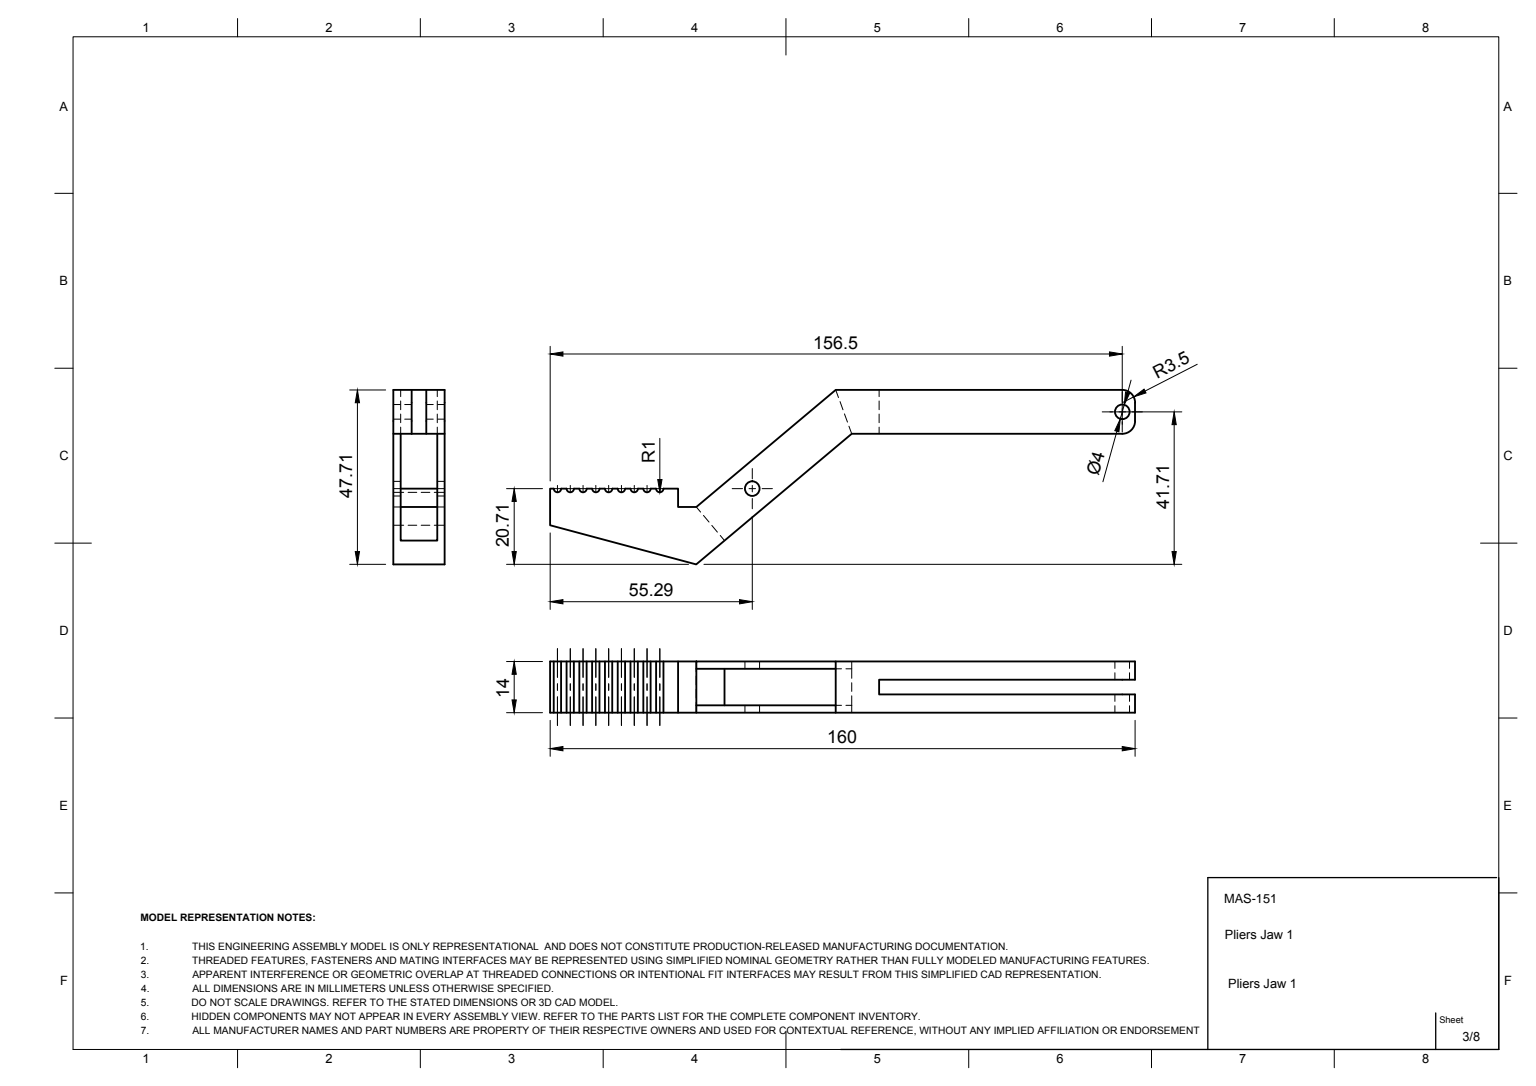
ISO-10303-21;
HEADER;
/* Generated by software containing ST-Developer
 * from STEP Tools, Inc. (www.steptools.com) 
 */

FILE_DESCRIPTION(
/* description */ ('STEP AP214'),
/* implementation_level */ '2;1');

FILE_NAME(
/* name */ 'Pliers Jaw 1.step',
/* time_stamp */ '2026-11-04T19:14:12-08:00',
/* author */ (''),
/* organization */ (''),
/* preprocessor_version */ 'ST-DEVELOPER v20.2',
/* originating_system */ 'Autodesk Translation Framework v15.17.0.0',
/* authorisation */ '');

FILE_SCHEMA (('AUTOMOTIVE_DESIGN { 1 0 10303 214 3 1 1 }'));
ENDSEC;

DATA;
#10=MECHANICAL_DESIGN_GEOMETRIC_PRESENTATION_REPRESENTATION('',(#99),#5990);
#85=SHAPE_REPRESENTATION_RELATIONSHIP('SRR','None',#6021,#92);
#92=ADVANCED_BREP_SHAPE_REPRESENTATION('',(#106),#5983);
#99=STYLED_ITEM('',(#6065),#106);
#106=MANIFOLD_SOLID_BREP('Body1',#3269);
#113=FACE_BOUND('',#427,.T.);
#114=FACE_BOUND('',#428,.T.);
#115=FACE_BOUND('',#430,.T.);
#116=FACE_BOUND('',#431,.T.);
#117=FACE_BOUND('',#463,.T.);
#118=FACE_BOUND('',#465,.T.);
#119=FACE_BOUND('',#467,.T.);
#120=FACE_BOUND('',#469,.T.);
#137=PLANE('',#3368);
#138=PLANE('',#3369);
#139=PLANE('',#3370);
#140=PLANE('',#3382);
#141=PLANE('',#3394);
#142=PLANE('',#3395);
#143=PLANE('',#3396);
#144=PLANE('',#3397);
#145=PLANE('',#3398);
#146=PLANE('',#3399);
#147=PLANE('',#3400);
#148=PLANE('',#3401);
#149=PLANE('',#3402);
#150=PLANE('',#3403);
#151=PLANE('',#3404);
#152=PLANE('',#3405);
#153=PLANE('',#3406);
#154=PLANE('',#3407);
#155=PLANE('',#3408);
#156=PLANE('',#3409);
#157=PLANE('',#3410);
#158=PLANE('',#3411);
#159=PLANE('',#3412);
#160=PLANE('',#3422);
#161=PLANE('',#3423);
#162=PLANE('',#3424);
#163=PLANE('',#3425);
#164=PLANE('',#3426);
#165=PLANE('',#3429);
#166=PLANE('',#3432);
#242=FACE_OUTER_BOUND('',#420,.T.);
#243=FACE_OUTER_BOUND('',#421,.T.);
#244=FACE_OUTER_BOUND('',#422,.T.);
#245=FACE_OUTER_BOUND('',#423,.T.);
#246=FACE_OUTER_BOUND('',#424,.T.);
#247=FACE_OUTER_BOUND('',#425,.T.);
#248=FACE_OUTER_BOUND('',#426,.T.);
#249=FACE_OUTER_BOUND('',#429,.T.);
#250=FACE_OUTER_BOUND('',#432,.T.);
#251=FACE_OUTER_BOUND('',#433,.T.);
#252=FACE_OUTER_BOUND('',#434,.T.);
#253=FACE_OUTER_BOUND('',#435,.T.);
#254=FACE_OUTER_BOUND('',#436,.T.);
#255=FACE_OUTER_BOUND('',#437,.T.);
#256=FACE_OUTER_BOUND('',#438,.T.);
#257=FACE_OUTER_BOUND('',#439,.T.);
#258=FACE_OUTER_BOUND('',#440,.T.);
#259=FACE_OUTER_BOUND('',#441,.T.);
#260=FACE_OUTER_BOUND('',#442,.T.);
#261=FACE_OUTER_BOUND('',#443,.T.);
#262=FACE_OUTER_BOUND('',#444,.T.);
#263=FACE_OUTER_BOUND('',#445,.T.);
#264=FACE_OUTER_BOUND('',#446,.T.);
#265=FACE_OUTER_BOUND('',#447,.T.);
#266=FACE_OUTER_BOUND('',#448,.T.);
#267=FACE_OUTER_BOUND('',#449,.T.);
#268=FACE_OUTER_BOUND('',#450,.T.);
#269=FACE_OUTER_BOUND('',#451,.T.);
#270=FACE_OUTER_BOUND('',#452,.T.);
#271=FACE_OUTER_BOUND('',#453,.T.);
#272=FACE_OUTER_BOUND('',#454,.T.);
#273=FACE_OUTER_BOUND('',#455,.T.);
#274=FACE_OUTER_BOUND('',#456,.T.);
#275=FACE_OUTER_BOUND('',#457,.T.);
#276=FACE_OUTER_BOUND('',#458,.T.);
#277=FACE_OUTER_BOUND('',#459,.T.);
#278=FACE_OUTER_BOUND('',#460,.T.);
#279=FACE_OUTER_BOUND('',#461,.T.);
#280=FACE_OUTER_BOUND('',#462,.T.);
#281=FACE_OUTER_BOUND('',#464,.T.);
#282=FACE_OUTER_BOUND('',#466,.T.);
#283=FACE_OUTER_BOUND('',#468,.T.);
#284=FACE_OUTER_BOUND('',#470,.T.);
#285=FACE_OUTER_BOUND('',#471,.T.);
#286=FACE_OUTER_BOUND('',#472,.T.);
#287=FACE_OUTER_BOUND('',#473,.T.);
#288=FACE_OUTER_BOUND('',#474,.T.);
#420=EDGE_LOOP('',(#2110,#2111,#2112,#2113));
#421=EDGE_LOOP('',(#2114,#2115,#2116,#2117));
#422=EDGE_LOOP('',(#2118,#2119,#2120,#2121));
#423=EDGE_LOOP('',(#2122,#2123,#2124,#2125));
#424=EDGE_LOOP('',(#2126,#2127,#2128,#2129));
#425=EDGE_LOOP('',(#2130,#2131,#2132,#2133));
#426=EDGE_LOOP('',(#2134,#2135,#2136,#2137,#2138,#2139,#2140,#2141,#2142,
#2143,#2144,#2145,#2146,#2147,#2148,#2149,#2150,#2151,#2152,#2153,#2154,
#2155,#2156,#2157,#2158,#2159,#2160,#2161,#2162,#2163));
#427=EDGE_LOOP('',(#2164));
#428=EDGE_LOOP('',(#2165));
#429=EDGE_LOOP('',(#2166,#2167,#2168,#2169,#2170,#2171,#2172,#2173,#2174,
#2175,#2176,#2177,#2178,#2179,#2180,#2181,#2182,#2183,#2184,#2185,#2186,
#2187,#2188,#2189,#2190,#2191,#2192,#2193,#2194,#2195));
#430=EDGE_LOOP('',(#2196));
#431=EDGE_LOOP('',(#2197));
#432=EDGE_LOOP('',(#2198,#2199,#2200,#2201));
#433=EDGE_LOOP('',(#2202,#2203,#2204,#2205));
#434=EDGE_LOOP('',(#2206,#2207,#2208,#2209));
#435=EDGE_LOOP('',(#2210,#2211,#2212,#2213));
#436=EDGE_LOOP('',(#2214,#2215,#2216,#2217));
#437=EDGE_LOOP('',(#2218,#2219,#2220,#2221));
#438=EDGE_LOOP('',(#2222,#2223,#2224,#2225));
#439=EDGE_LOOP('',(#2226,#2227,#2228,#2229));
#440=EDGE_LOOP('',(#2230,#2231,#2232,#2233));
#441=EDGE_LOOP('',(#2234,#2235,#2236,#2237,#2238,#2239));
#442=EDGE_LOOP('',(#2240,#2241,#2242,#2243));
#443=EDGE_LOOP('',(#2244,#2245,#2246,#2247));
#444=EDGE_LOOP('',(#2248,#2249,#2250,#2251));
#445=EDGE_LOOP('',(#2252,#2253,#2254,#2255,#2256,#2257,#2258,#2259));
#446=EDGE_LOOP('',(#2260,#2261,#2262,#2263,#2264,#2265,#2266,#2267,#2268,
#2269));
#447=EDGE_LOOP('',(#2270,#2271,#2272,#2273));
#448=EDGE_LOOP('',(#2274,#2275,#2276,#2277,#2278,#2279,#2280,#2281,#2282,
#2283));
#449=EDGE_LOOP('',(#2284,#2285,#2286,#2287));
#450=EDGE_LOOP('',(#2288,#2289,#2290,#2291));
#451=EDGE_LOOP('',(#2292,#2293,#2294,#2295));
#452=EDGE_LOOP('',(#2296,#2297,#2298,#2299));
#453=EDGE_LOOP('',(#2300,#2301,#2302,#2303));
#454=EDGE_LOOP('',(#2304,#2305,#2306,#2307));
#455=EDGE_LOOP('',(#2308,#2309,#2310,#2311));
#456=EDGE_LOOP('',(#2312,#2313,#2314,#2315));
#457=EDGE_LOOP('',(#2316,#2317,#2318,#2319));
#458=EDGE_LOOP('',(#2320,#2321,#2322,#2323));
#459=EDGE_LOOP('',(#2324,#2325,#2326,#2327));
#460=EDGE_LOOP('',(#2328,#2329,#2330,#2331));
#461=EDGE_LOOP('',(#2332,#2333,#2334,#2335));
#462=EDGE_LOOP('',(#2336,#2337,#2338,#2339));
#463=EDGE_LOOP('',(#2340));
#464=EDGE_LOOP('',(#2341,#2342,#2343,#2344));
#465=EDGE_LOOP('',(#2345));
#466=EDGE_LOOP('',(#2346,#2347,#2348,#2349,#2350,#2351));
#467=EDGE_LOOP('',(#2352));
#468=EDGE_LOOP('',(#2353,#2354,#2355,#2356,#2357,#2358));
#469=EDGE_LOOP('',(#2359));
#470=EDGE_LOOP('',(#2360,#2361,#2362,#2363));
#471=EDGE_LOOP('',(#2364,#2365,#2366,#2367));
#472=EDGE_LOOP('',(#2368,#2369,#2370,#2371));
#473=EDGE_LOOP('',(#2372,#2373,#2374,#2375));
#474=EDGE_LOOP('',(#2376,#2377,#2378,#2379));
#622=LINE('',#4656,#925);
#623=LINE('',#4662,#926);
#624=LINE('',#4668,#927);
#625=LINE('',#4674,#928);
#626=LINE('',#4679,#929);
#627=LINE('',#4681,#930);
#628=LINE('',#4683,#931);
#629=LINE('',#4684,#932);
#630=LINE('',#4688,#933);
#631=LINE('',#4690,#934);
#632=LINE('',#4692,#935);
#633=LINE('',#4693,#936);
#634=LINE('',#4697,#937);
#635=LINE('',#4701,#938);
#636=LINE('',#4703,#939);
#637=LINE('',#4705,#940);
#638=LINE('',#4707,#941);
#639=LINE('',#4709,#942);
#640=LINE('',#4713,#943);
#641=LINE('',#4717,#944);
#642=LINE('',#4721,#945);
#643=LINE('',#4725,#946);
#644=LINE('',#4729,#947);
#645=LINE('',#4733,#948);
#646=LINE('',#4737,#949);
#647=LINE('',#4741,#950);
#648=LINE('',#4745,#951);
#649=LINE('',#4747,#952);
#650=LINE('',#4749,#953);
#651=LINE('',#4751,#954);
#652=LINE('',#4753,#955);
#653=LINE('',#4757,#956);
#654=LINE('',#4762,#957);
#655=LINE('',#4764,#958);
#656=LINE('',#4766,#959);
#657=LINE('',#4768,#960);
#658=LINE('',#4770,#961);
#659=LINE('',#4774,#962);
#660=LINE('',#4778,#963);
#661=LINE('',#4782,#964);
#662=LINE('',#4786,#965);
#663=LINE('',#4790,#966);
#664=LINE('',#4794,#967);
#665=LINE('',#4798,#968);
#666=LINE('',#4802,#969);
#667=LINE('',#4806,#970);
#668=LINE('',#4808,#971);
#669=LINE('',#4809,#972);
#670=LINE('',#4811,#973);
#671=LINE('',#4812,#974);
#672=LINE('',#4814,#975);
#673=LINE('',#4815,#976);
#674=LINE('',#4817,#977);
#675=LINE('',#4818,#978);
#676=LINE('',#4820,#979);
#677=LINE('',#4821,#980);
#678=LINE('',#4823,#981);
#679=LINE('',#4824,#982);
#680=LINE('',#4826,#983);
#681=LINE('',#4827,#984);
#682=LINE('',#4829,#985);
#683=LINE('',#4830,#986);
#684=LINE('',#4832,#987);
#685=LINE('',#4833,#988);
#686=LINE('',#4835,#989);
#687=LINE('',#4836,#990);
#688=LINE('',#4838,#991);
#689=LINE('',#4840,#992);
#690=LINE('',#4841,#993);
#691=LINE('',#4844,#994);
#692=LINE('',#4845,#995);
#693=LINE('',#4847,#996);
#694=LINE('',#4848,#997);
#695=LINE('',#4850,#998);
#696=LINE('',#4854,#999);
#697=LINE('',#4856,#1000);
#698=LINE('',#4857,#1001);
#699=LINE('',#4859,#1002);
#700=LINE('',#4860,#1003);
#701=LINE('',#4864,#1004);
#702=LINE('',#4865,#1005);
#703=LINE('',#4866,#1006);
#704=LINE('',#4868,#1007);
#705=LINE('',#4870,#1008);
#706=LINE('',#4871,#1009);
#707=LINE('',#4875,#1010);
#708=LINE('',#4876,#1011);
#709=LINE('',#4877,#1012);
#710=LINE('',#4880,#1013);
#711=LINE('',#4882,#1014);
#712=LINE('',#4884,#1015);
#713=LINE('',#4886,#1016);
#714=LINE('',#4887,#1017);
#715=LINE('',#4888,#1018);
#716=LINE('',#4891,#1019);
#717=LINE('',#4902,#1020);
#718=LINE('',#4903,#1021);
#719=LINE('',#4905,#1022);
#720=LINE('',#4906,#1023);
#721=LINE('',#4912,#1024);
#722=LINE('',#4915,#1025);
#925=VECTOR('',#3693,2.);
#926=VECTOR('',#3700,2.);
#927=VECTOR('',#3707,2.);
#928=VECTOR('',#3714,2.);
#929=VECTOR('',#3719,1000.);
#930=VECTOR('',#3720,1000.);
#931=VECTOR('',#3721,1000.);
#932=VECTOR('',#3722,1000.);
#933=VECTOR('',#3725,1000.);
#934=VECTOR('',#3726,1000.);
#935=VECTOR('',#3727,1000.);
#936=VECTOR('',#3728,1000.);
#937=VECTOR('',#3731,1000.);
#938=VECTOR('',#3734,1000.);
#939=VECTOR('',#3735,1000.);
#940=VECTOR('',#3736,1000.);
#941=VECTOR('',#3737,1000.);
#942=VECTOR('',#3738,1000.);
#943=VECTOR('',#3741,1000.);
#944=VECTOR('',#3744,1000.);
#945=VECTOR('',#3747,1000.);
#946=VECTOR('',#3750,1000.);
#947=VECTOR('',#3753,1000.);
#948=VECTOR('',#3756,1000.);
#949=VECTOR('',#3759,1000.);
#950=VECTOR('',#3762,1000.);
#951=VECTOR('',#3765,1000.);
#952=VECTOR('',#3766,1000.);
#953=VECTOR('',#3767,1000.);
#954=VECTOR('',#3768,1000.);
#955=VECTOR('',#3769,1000.);
#956=VECTOR('',#3774,1000.);
#957=VECTOR('',#3779,1000.);
#958=VECTOR('',#3780,1000.);
#959=VECTOR('',#3781,1000.);
#960=VECTOR('',#3782,1000.);
#961=VECTOR('',#3783,1000.);
#962=VECTOR('',#3786,1000.);
#963=VECTOR('',#3789,1000.);
#964=VECTOR('',#3792,1000.);
#965=VECTOR('',#3795,1000.);
#966=VECTOR('',#3798,1000.);
#967=VECTOR('',#3801,1000.);
#968=VECTOR('',#3804,1000.);
#969=VECTOR('',#3807,1000.);
#970=VECTOR('',#3810,1000.);
#971=VECTOR('',#3811,1000.);
#972=VECTOR('',#3812,1000.);
#973=VECTOR('',#3815,1000.);
#974=VECTOR('',#3816,1000.);
#975=VECTOR('',#3819,1000.);
#976=VECTOR('',#3820,1000.);
#977=VECTOR('',#3823,1000.);
#978=VECTOR('',#3824,1000.);
#979=VECTOR('',#3827,1000.);
#980=VECTOR('',#3828,1000.);
#981=VECTOR('',#3831,1000.);
#982=VECTOR('',#3832,1000.);
#983=VECTOR('',#3835,1000.);
#984=VECTOR('',#3836,1000.);
#985=VECTOR('',#3839,1000.);
#986=VECTOR('',#3840,1000.);
#987=VECTOR('',#3843,1000.);
#988=VECTOR('',#3844,1000.);
#989=VECTOR('',#3847,1000.);
#990=VECTOR('',#3848,1000.);
#991=VECTOR('',#3851,1000.);
#992=VECTOR('',#3852,1000.);
#993=VECTOR('',#3853,1000.);
#994=VECTOR('',#3856,1000.);
#995=VECTOR('',#3857,1000.);
#996=VECTOR('',#3860,1000.);
#997=VECTOR('',#3861,1000.);
#998=VECTOR('',#3864,1000.);
#999=VECTOR('',#3867,1000.);
#1000=VECTOR('',#3868,1000.);
#1001=VECTOR('',#3869,1000.);
#1002=VECTOR('',#3870,1000.);
#1003=VECTOR('',#3871,1000.);
#1004=VECTOR('',#3874,1000.);
#1005=VECTOR('',#3875,1000.);
#1006=VECTOR('',#3876,1000.);
#1007=VECTOR('',#3877,1000.);
#1008=VECTOR('',#3878,1000.);
#1009=VECTOR('',#3879,1000.);
#1010=VECTOR('',#3882,1000.);
#1011=VECTOR('',#3883,1000.);
#1012=VECTOR('',#3884,1000.);
#1013=VECTOR('',#3887,1000.);
#1014=VECTOR('',#3888,1000.);
#1015=VECTOR('',#3889,1000.);
#1016=VECTOR('',#3890,1000.);
#1017=VECTOR('',#3891,1000.);
#1018=VECTOR('',#3892,1000.);
#1019=VECTOR('',#3897,1000.);
#1020=VECTOR('',#3918,1000.);
#1021=VECTOR('',#3919,1000.);
#1022=VECTOR('',#3922,1000.);
#1023=VECTOR('',#3923,1000.);
#1024=VECTOR('',#3934,1000.);
#1025=VECTOR('',#3939,1000.);
#1228=CIRCLE('',#3357,2.);
#1229=CIRCLE('',#3358,2.);
#1230=CIRCLE('',#3360,2.);
#1231=CIRCLE('',#3361,2.);
#1232=CIRCLE('',#3363,2.);
#1233=CIRCLE('',#3364,2.);
#1234=CIRCLE('',#3366,2.);
#1235=CIRCLE('',#3367,2.);
#1236=CIRCLE('',#3371,3.5);
#1237=CIRCLE('',#3372,1.);
#1238=CIRCLE('',#3373,1.);
#1239=CIRCLE('',#3374,1.);
#1240=CIRCLE('',#3375,1.);
#1241=CIRCLE('',#3376,1.);
#1242=CIRCLE('',#3377,1.);
#1243=CIRCLE('',#3378,1.);
#1244=CIRCLE('',#3379,1.);
#1245=CIRCLE('',#3380,1.);
#1246=CIRCLE('',#3381,3.5);
#1247=CIRCLE('',#3383,3.5);
#1248=CIRCLE('',#3384,3.5);
#1249=CIRCLE('',#3385,1.);
#1250=CIRCLE('',#3386,1.);
#1251=CIRCLE('',#3387,1.);
#1252=CIRCLE('',#3388,1.);
#1253=CIRCLE('',#3389,1.);
#1254=CIRCLE('',#3390,1.);
#1255=CIRCLE('',#3391,1.);
#1256=CIRCLE('',#3392,1.);
#1257=CIRCLE('',#3393,1.);
#1258=CIRCLE('',#3427,3.5);
#1259=CIRCLE('',#3428,3.5);
#1260=CIRCLE('',#3430,3.5);
#1261=CIRCLE('',#3431,3.5);
#1356=VERTEX_POINT('',#4653);
#1357=VERTEX_POINT('',#4655);
#1358=VERTEX_POINT('',#4659);
#1359=VERTEX_POINT('',#4661);
#1360=VERTEX_POINT('',#4665);
#1361=VERTEX_POINT('',#4667);
#1362=VERTEX_POINT('',#4671);
#1363=VERTEX_POINT('',#4673);
#1364=VERTEX_POINT('',#4677);
#1365=VERTEX_POINT('',#4678);
#1366=VERTEX_POINT('',#4680);
#1367=VERTEX_POINT('',#4682);
#1368=VERTEX_POINT('',#4686);
#1369=VERTEX_POINT('',#4687);
#1370=VERTEX_POINT('',#4689);
#1371=VERTEX_POINT('',#4691);
#1372=VERTEX_POINT('',#4695);
#1373=VERTEX_POINT('',#4696);
#1374=VERTEX_POINT('',#4698);
#1375=VERTEX_POINT('',#4700);
#1376=VERTEX_POINT('',#4702);
#1377=VERTEX_POINT('',#4704);
#1378=VERTEX_POINT('',#4706);
#1379=VERTEX_POINT('',#4708);
#1380=VERTEX_POINT('',#4710);
#1381=VERTEX_POINT('',#4712);
#1382=VERTEX_POINT('',#4714);
#1383=VERTEX_POINT('',#4716);
#1384=VERTEX_POINT('',#4718);
#1385=VERTEX_POINT('',#4720);
#1386=VERTEX_POINT('',#4722);
#1387=VERTEX_POINT('',#4724);
#1388=VERTEX_POINT('',#4726);
#1389=VERTEX_POINT('',#4728);
#1390=VERTEX_POINT('',#4730);
#1391=VERTEX_POINT('',#4732);
#1392=VERTEX_POINT('',#4734);
#1393=VERTEX_POINT('',#4736);
#1394=VERTEX_POINT('',#4738);
#1395=VERTEX_POINT('',#4740);
#1396=VERTEX_POINT('',#4742);
#1397=VERTEX_POINT('',#4744);
#1398=VERTEX_POINT('',#4746);
#1399=VERTEX_POINT('',#4748);
#1400=VERTEX_POINT('',#4750);
#1401=VERTEX_POINT('',#4752);
#1402=VERTEX_POINT('',#4756);
#1403=VERTEX_POINT('',#4759);
#1404=VERTEX_POINT('',#4761);
#1405=VERTEX_POINT('',#4763);
#1406=VERTEX_POINT('',#4765);
#1407=VERTEX_POINT('',#4767);
#1408=VERTEX_POINT('',#4769);
#1409=VERTEX_POINT('',#4771);
#1410=VERTEX_POINT('',#4773);
#1411=VERTEX_POINT('',#4775);
#1412=VERTEX_POINT('',#4777);
#1413=VERTEX_POINT('',#4779);
#1414=VERTEX_POINT('',#4781);
#1415=VERTEX_POINT('',#4783);
#1416=VERTEX_POINT('',#4785);
#1417=VERTEX_POINT('',#4787);
#1418=VERTEX_POINT('',#4789);
#1419=VERTEX_POINT('',#4791);
#1420=VERTEX_POINT('',#4793);
#1421=VERTEX_POINT('',#4795);
#1422=VERTEX_POINT('',#4797);
#1423=VERTEX_POINT('',#4799);
#1424=VERTEX_POINT('',#4801);
#1425=VERTEX_POINT('',#4803);
#1426=VERTEX_POINT('',#4805);
#1427=VERTEX_POINT('',#4807);
#1428=VERTEX_POINT('',#4839);
#1429=VERTEX_POINT('',#4843);
#1430=VERTEX_POINT('',#4852);
#1431=VERTEX_POINT('',#4853);
#1432=VERTEX_POINT('',#4855);
#1433=VERTEX_POINT('',#4858);
#1434=VERTEX_POINT('',#4862);
#1435=VERTEX_POINT('',#4863);
#1436=VERTEX_POINT('',#4867);
#1437=VERTEX_POINT('',#4869);
#1438=VERTEX_POINT('',#4873);
#1439=VERTEX_POINT('',#4874);
#1440=VERTEX_POINT('',#4879);
#1441=VERTEX_POINT('',#4881);
#1442=VERTEX_POINT('',#4883);
#1443=VERTEX_POINT('',#4885);
#1651=EDGE_CURVE('',#1356,#1356,#1228,.T.);
#1652=EDGE_CURVE('',#1356,#1357,#622,.T.);
#1653=EDGE_CURVE('',#1357,#1357,#1229,.T.);
#1654=EDGE_CURVE('',#1358,#1358,#1230,.T.);
#1655=EDGE_CURVE('',#1358,#1359,#623,.T.);
#1656=EDGE_CURVE('',#1359,#1359,#1231,.T.);
#1657=EDGE_CURVE('',#1360,#1360,#1232,.T.);
#1658=EDGE_CURVE('',#1360,#1361,#624,.T.);
#1659=EDGE_CURVE('',#1361,#1361,#1233,.T.);
#1660=EDGE_CURVE('',#1362,#1362,#1234,.T.);
#1661=EDGE_CURVE('',#1362,#1363,#625,.T.);
#1662=EDGE_CURVE('',#1363,#1363,#1235,.T.);
#1663=EDGE_CURVE('',#1364,#1365,#626,.T.);
#1664=EDGE_CURVE('',#1365,#1366,#627,.T.);
#1665=EDGE_CURVE('',#1366,#1367,#628,.T.);
#1666=EDGE_CURVE('',#1367,#1364,#629,.T.);
#1667=EDGE_CURVE('',#1368,#1369,#630,.T.);
#1668=EDGE_CURVE('',#1368,#1370,#631,.T.);
#1669=EDGE_CURVE('',#1370,#1371,#632,.T.);
#1670=EDGE_CURVE('',#1369,#1371,#633,.T.);
#1671=EDGE_CURVE('',#1372,#1373,#634,.T.);
#1672=EDGE_CURVE('',#1373,#1374,#1236,.T.);
#1673=EDGE_CURVE('',#1374,#1375,#635,.T.);
#1674=EDGE_CURVE('',#1375,#1376,#636,.T.);
#1675=EDGE_CURVE('',#1376,#1377,#637,.T.);
#1676=EDGE_CURVE('',#1377,#1378,#638,.T.);
#1677=EDGE_CURVE('',#1378,#1379,#639,.T.);
#1678=EDGE_CURVE('',#1380,#1379,#1237,.T.);
#1679=EDGE_CURVE('',#1380,#1381,#640,.T.);
#1680=EDGE_CURVE('',#1382,#1381,#1238,.T.);
#1681=EDGE_CURVE('',#1382,#1383,#641,.T.);
#1682=EDGE_CURVE('',#1384,#1383,#1239,.T.);
#1683=EDGE_CURVE('',#1384,#1385,#642,.T.);
#1684=EDGE_CURVE('',#1386,#1385,#1240,.T.);
#1685=EDGE_CURVE('',#1386,#1387,#643,.T.);
#1686=EDGE_CURVE('',#1388,#1387,#1241,.T.);
#1687=EDGE_CURVE('',#1388,#1389,#644,.T.);
#1688=EDGE_CURVE('',#1390,#1389,#1242,.T.);
#1689=EDGE_CURVE('',#1390,#1391,#645,.T.);
#1690=EDGE_CURVE('',#1392,#1391,#1243,.T.);
#1691=EDGE_CURVE('',#1392,#1393,#646,.T.);
#1692=EDGE_CURVE('',#1394,#1393,#1244,.T.);
#1693=EDGE_CURVE('',#1394,#1395,#647,.T.);
#1694=EDGE_CURVE('',#1396,#1395,#1245,.T.);
#1695=EDGE_CURVE('',#1396,#1397,#648,.T.);
#1696=EDGE_CURVE('',#1397,#1398,#649,.T.);
#1697=EDGE_CURVE('',#1398,#1399,#650,.T.);
#1698=EDGE_CURVE('',#1399,#1400,#651,.T.);
#1699=EDGE_CURVE('',#1400,#1401,#652,.T.);
#1700=EDGE_CURVE('',#1401,#1372,#1246,.T.);
#1701=EDGE_CURVE('',#1402,#1370,#653,.T.);
#1702=EDGE_CURVE('',#1402,#1365,#1247,.T.);
#1703=EDGE_CURVE('',#1364,#1403,#1248,.T.);
#1704=EDGE_CURVE('',#1404,#1403,#654,.T.);
#1705=EDGE_CURVE('',#1405,#1404,#655,.T.);
#1706=EDGE_CURVE('',#1406,#1405,#656,.T.);
#1707=EDGE_CURVE('',#1407,#1406,#657,.T.);
#1708=EDGE_CURVE('',#1408,#1407,#658,.T.);
#1709=EDGE_CURVE('',#1408,#1409,#1249,.T.);
#1710=EDGE_CURVE('',#1410,#1409,#659,.T.);
#1711=EDGE_CURVE('',#1410,#1411,#1250,.T.);
#1712=EDGE_CURVE('',#1412,#1411,#660,.T.);
#1713=EDGE_CURVE('',#1412,#1413,#1251,.T.);
#1714=EDGE_CURVE('',#1414,#1413,#661,.T.);
#1715=EDGE_CURVE('',#1414,#1415,#1252,.T.);
#1716=EDGE_CURVE('',#1416,#1415,#662,.T.);
#1717=EDGE_CURVE('',#1416,#1417,#1253,.T.);
#1718=EDGE_CURVE('',#1418,#1417,#663,.T.);
#1719=EDGE_CURVE('',#1418,#1419,#1254,.T.);
#1720=EDGE_CURVE('',#1420,#1419,#664,.T.);
#1721=EDGE_CURVE('',#1420,#1421,#1255,.T.);
#1722=EDGE_CURVE('',#1422,#1421,#665,.T.);
#1723=EDGE_CURVE('',#1422,#1423,#1256,.T.);
#1724=EDGE_CURVE('',#1424,#1423,#666,.T.);
#1725=EDGE_CURVE('',#1424,#1425,#1257,.T.);
#1726=EDGE_CURVE('',#1426,#1425,#667,.T.);
#1727=EDGE_CURVE('',#1427,#1426,#668,.T.);
#1728=EDGE_CURVE('',#1371,#1427,#669,.T.);
#1729=EDGE_CURVE('',#1411,#1393,#670,.T.);
#1730=EDGE_CURVE('',#1392,#1412,#671,.T.);
#1731=EDGE_CURVE('',#1413,#1391,#672,.T.);
#1732=EDGE_CURVE('',#1390,#1414,#673,.T.);
#1733=EDGE_CURVE('',#1415,#1389,#674,.T.);
#1734=EDGE_CURVE('',#1388,#1416,#675,.T.);
#1735=EDGE_CURVE('',#1417,#1387,#676,.T.);
#1736=EDGE_CURVE('',#1386,#1418,#677,.T.);
#1737=EDGE_CURVE('',#1419,#1385,#678,.T.);
#1738=EDGE_CURVE('',#1384,#1420,#679,.T.);
#1739=EDGE_CURVE('',#1421,#1383,#680,.T.);
#1740=EDGE_CURVE('',#1382,#1422,#681,.T.);
#1741=EDGE_CURVE('',#1423,#1381,#682,.T.);
#1742=EDGE_CURVE('',#1380,#1424,#683,.T.);
#1743=EDGE_CURVE('',#1425,#1379,#684,.T.);
#1744=EDGE_CURVE('',#1378,#1426,#685,.T.);
#1745=EDGE_CURVE('',#1394,#1410,#686,.T.);
#1746=EDGE_CURVE('',#1409,#1395,#687,.T.);
#1747=EDGE_CURVE('',#1377,#1427,#688,.T.);
#1748=EDGE_CURVE('',#1376,#1428,#689,.T.);
#1749=EDGE_CURVE('',#1369,#1428,#690,.T.);
#1750=EDGE_CURVE('',#1375,#1429,#691,.T.);
#1751=EDGE_CURVE('',#1429,#1428,#692,.T.);
#1752=EDGE_CURVE('',#1398,#1406,#693,.T.);
#1753=EDGE_CURVE('',#1397,#1407,#694,.T.);
#1754=EDGE_CURVE('',#1399,#1405,#695,.T.);
#1755=EDGE_CURVE('',#1430,#1431,#696,.T.);
#1756=EDGE_CURVE('',#1431,#1432,#697,.T.);
#1757=EDGE_CURVE('',#1400,#1432,#698,.T.);
#1758=EDGE_CURVE('',#1433,#1404,#699,.T.);
#1759=EDGE_CURVE('',#1430,#1433,#700,.T.);
#1760=EDGE_CURVE('',#1434,#1435,#701,.T.);
#1761=EDGE_CURVE('',#1435,#1401,#702,.T.);
#1762=EDGE_CURVE('',#1433,#1432,#703,.T.);
#1763=EDGE_CURVE('',#1403,#1436,#704,.T.);
#1764=EDGE_CURVE('',#1437,#1436,#705,.T.);
#1765=EDGE_CURVE('',#1434,#1437,#706,.T.);
#1766=EDGE_CURVE('',#1438,#1439,#707,.T.);
#1767=EDGE_CURVE('',#1438,#1373,#708,.T.);
#1768=EDGE_CURVE('',#1372,#1439,#709,.T.);
#1769=EDGE_CURVE('',#1374,#1440,#710,.T.);
#1770=EDGE_CURVE('',#1440,#1441,#711,.T.);
#1771=EDGE_CURVE('',#1442,#1441,#712,.T.);
#1772=EDGE_CURVE('',#1443,#1442,#713,.T.);
#1773=EDGE_CURVE('',#1443,#1402,#714,.T.);
#1774=EDGE_CURVE('',#1368,#1429,#715,.T.);
#1775=EDGE_CURVE('',#1396,#1408,#716,.T.);
#1776=EDGE_CURVE('',#1432,#1429,#717,.T.);
#1777=EDGE_CURVE('',#1433,#1368,#718,.T.);
#1778=EDGE_CURVE('',#1428,#1431,#719,.T.);
#1779=EDGE_CURVE('',#1369,#1430,#720,.T.);
#1780=EDGE_CURVE('',#1440,#1438,#1258,.T.);
#1781=EDGE_CURVE('',#1439,#1435,#1259,.T.);
#1782=EDGE_CURVE('',#1441,#1434,#721,.T.);
#1783=EDGE_CURVE('',#1366,#1443,#1260,.T.);
#1784=EDGE_CURVE('',#1442,#1437,#722,.T.);
#1785=EDGE_CURVE('',#1436,#1367,#1261,.T.);
#2110=ORIENTED_EDGE('',*,*,#1651,.F.);
#2111=ORIENTED_EDGE('',*,*,#1652,.T.);
#2112=ORIENTED_EDGE('',*,*,#1653,.F.);
#2113=ORIENTED_EDGE('',*,*,#1652,.F.);
#2114=ORIENTED_EDGE('',*,*,#1654,.T.);
#2115=ORIENTED_EDGE('',*,*,#1655,.T.);
#2116=ORIENTED_EDGE('',*,*,#1656,.T.);
#2117=ORIENTED_EDGE('',*,*,#1655,.F.);
#2118=ORIENTED_EDGE('',*,*,#1657,.F.);
#2119=ORIENTED_EDGE('',*,*,#1658,.T.);
#2120=ORIENTED_EDGE('',*,*,#1659,.T.);
#2121=ORIENTED_EDGE('',*,*,#1658,.F.);
#2122=ORIENTED_EDGE('',*,*,#1660,.F.);
#2123=ORIENTED_EDGE('',*,*,#1661,.T.);
#2124=ORIENTED_EDGE('',*,*,#1662,.T.);
#2125=ORIENTED_EDGE('',*,*,#1661,.F.);
#2126=ORIENTED_EDGE('',*,*,#1663,.T.);
#2127=ORIENTED_EDGE('',*,*,#1664,.T.);
#2128=ORIENTED_EDGE('',*,*,#1665,.T.);
#2129=ORIENTED_EDGE('',*,*,#1666,.T.);
#2130=ORIENTED_EDGE('',*,*,#1667,.F.);
#2131=ORIENTED_EDGE('',*,*,#1668,.T.);
#2132=ORIENTED_EDGE('',*,*,#1669,.T.);
#2133=ORIENTED_EDGE('',*,*,#1670,.F.);
#2134=ORIENTED_EDGE('',*,*,#1671,.T.);
#2135=ORIENTED_EDGE('',*,*,#1672,.T.);
#2136=ORIENTED_EDGE('',*,*,#1673,.T.);
#2137=ORIENTED_EDGE('',*,*,#1674,.T.);
#2138=ORIENTED_EDGE('',*,*,#1675,.T.);
#2139=ORIENTED_EDGE('',*,*,#1676,.T.);
#2140=ORIENTED_EDGE('',*,*,#1677,.T.);
#2141=ORIENTED_EDGE('',*,*,#1678,.F.);
#2142=ORIENTED_EDGE('',*,*,#1679,.T.);
#2143=ORIENTED_EDGE('',*,*,#1680,.F.);
#2144=ORIENTED_EDGE('',*,*,#1681,.T.);
#2145=ORIENTED_EDGE('',*,*,#1682,.F.);
#2146=ORIENTED_EDGE('',*,*,#1683,.T.);
#2147=ORIENTED_EDGE('',*,*,#1684,.F.);
#2148=ORIENTED_EDGE('',*,*,#1685,.T.);
#2149=ORIENTED_EDGE('',*,*,#1686,.F.);
#2150=ORIENTED_EDGE('',*,*,#1687,.T.);
#2151=ORIENTED_EDGE('',*,*,#1688,.F.);
#2152=ORIENTED_EDGE('',*,*,#1689,.T.);
#2153=ORIENTED_EDGE('',*,*,#1690,.F.);
#2154=ORIENTED_EDGE('',*,*,#1691,.T.);
#2155=ORIENTED_EDGE('',*,*,#1692,.F.);
#2156=ORIENTED_EDGE('',*,*,#1693,.T.);
#2157=ORIENTED_EDGE('',*,*,#1694,.F.);
#2158=ORIENTED_EDGE('',*,*,#1695,.T.);
#2159=ORIENTED_EDGE('',*,*,#1696,.T.);
#2160=ORIENTED_EDGE('',*,*,#1697,.T.);
#2161=ORIENTED_EDGE('',*,*,#1698,.T.);
#2162=ORIENTED_EDGE('',*,*,#1699,.T.);
#2163=ORIENTED_EDGE('',*,*,#1700,.T.);
#2164=ORIENTED_EDGE('',*,*,#1651,.T.);
#2165=ORIENTED_EDGE('',*,*,#1662,.F.);
#2166=ORIENTED_EDGE('',*,*,#1701,.F.);
#2167=ORIENTED_EDGE('',*,*,#1702,.T.);
#2168=ORIENTED_EDGE('',*,*,#1663,.F.);
#2169=ORIENTED_EDGE('',*,*,#1703,.T.);
#2170=ORIENTED_EDGE('',*,*,#1704,.F.);
#2171=ORIENTED_EDGE('',*,*,#1705,.F.);
#2172=ORIENTED_EDGE('',*,*,#1706,.F.);
#2173=ORIENTED_EDGE('',*,*,#1707,.F.);
#2174=ORIENTED_EDGE('',*,*,#1708,.F.);
#2175=ORIENTED_EDGE('',*,*,#1709,.T.);
#2176=ORIENTED_EDGE('',*,*,#1710,.F.);
#2177=ORIENTED_EDGE('',*,*,#1711,.T.);
#2178=ORIENTED_EDGE('',*,*,#1712,.F.);
#2179=ORIENTED_EDGE('',*,*,#1713,.T.);
#2180=ORIENTED_EDGE('',*,*,#1714,.F.);
#2181=ORIENTED_EDGE('',*,*,#1715,.T.);
#2182=ORIENTED_EDGE('',*,*,#1716,.F.);
#2183=ORIENTED_EDGE('',*,*,#1717,.T.);
#2184=ORIENTED_EDGE('',*,*,#1718,.F.);
#2185=ORIENTED_EDGE('',*,*,#1719,.T.);
#2186=ORIENTED_EDGE('',*,*,#1720,.F.);
#2187=ORIENTED_EDGE('',*,*,#1721,.T.);
#2188=ORIENTED_EDGE('',*,*,#1722,.F.);
#2189=ORIENTED_EDGE('',*,*,#1723,.T.);
#2190=ORIENTED_EDGE('',*,*,#1724,.F.);
#2191=ORIENTED_EDGE('',*,*,#1725,.T.);
#2192=ORIENTED_EDGE('',*,*,#1726,.F.);
#2193=ORIENTED_EDGE('',*,*,#1727,.F.);
#2194=ORIENTED_EDGE('',*,*,#1728,.F.);
#2195=ORIENTED_EDGE('',*,*,#1669,.F.);
#2196=ORIENTED_EDGE('',*,*,#1656,.F.);
#2197=ORIENTED_EDGE('',*,*,#1657,.T.);
#2198=ORIENTED_EDGE('',*,*,#1712,.T.);
#2199=ORIENTED_EDGE('',*,*,#1729,.T.);
#2200=ORIENTED_EDGE('',*,*,#1691,.F.);
#2201=ORIENTED_EDGE('',*,*,#1730,.T.);
#2202=ORIENTED_EDGE('',*,*,#1714,.T.);
#2203=ORIENTED_EDGE('',*,*,#1731,.T.);
#2204=ORIENTED_EDGE('',*,*,#1689,.F.);
#2205=ORIENTED_EDGE('',*,*,#1732,.T.);
#2206=ORIENTED_EDGE('',*,*,#1716,.T.);
#2207=ORIENTED_EDGE('',*,*,#1733,.T.);
#2208=ORIENTED_EDGE('',*,*,#1687,.F.);
#2209=ORIENTED_EDGE('',*,*,#1734,.T.);
#2210=ORIENTED_EDGE('',*,*,#1718,.T.);
#2211=ORIENTED_EDGE('',*,*,#1735,.T.);
#2212=ORIENTED_EDGE('',*,*,#1685,.F.);
#2213=ORIENTED_EDGE('',*,*,#1736,.T.);
#2214=ORIENTED_EDGE('',*,*,#1720,.T.);
#2215=ORIENTED_EDGE('',*,*,#1737,.T.);
#2216=ORIENTED_EDGE('',*,*,#1683,.F.);
#2217=ORIENTED_EDGE('',*,*,#1738,.T.);
#2218=ORIENTED_EDGE('',*,*,#1722,.T.);
#2219=ORIENTED_EDGE('',*,*,#1739,.T.);
#2220=ORIENTED_EDGE('',*,*,#1681,.F.);
#2221=ORIENTED_EDGE('',*,*,#1740,.T.);
#2222=ORIENTED_EDGE('',*,*,#1724,.T.);
#2223=ORIENTED_EDGE('',*,*,#1741,.T.);
#2224=ORIENTED_EDGE('',*,*,#1679,.F.);
#2225=ORIENTED_EDGE('',*,*,#1742,.T.);
#2226=ORIENTED_EDGE('',*,*,#1726,.T.);
#2227=ORIENTED_EDGE('',*,*,#1743,.T.);
#2228=ORIENTED_EDGE('',*,*,#1677,.F.);
#2229=ORIENTED_EDGE('',*,*,#1744,.T.);
#2230=ORIENTED_EDGE('',*,*,#1693,.F.);
#2231=ORIENTED_EDGE('',*,*,#1745,.T.);
#2232=ORIENTED_EDGE('',*,*,#1710,.T.);
#2233=ORIENTED_EDGE('',*,*,#1746,.T.);
#2234=ORIENTED_EDGE('',*,*,#1747,.F.);
#2235=ORIENTED_EDGE('',*,*,#1675,.F.);
#2236=ORIENTED_EDGE('',*,*,#1748,.T.);
#2237=ORIENTED_EDGE('',*,*,#1749,.F.);
#2238=ORIENTED_EDGE('',*,*,#1670,.T.);
#2239=ORIENTED_EDGE('',*,*,#1728,.T.);
#2240=ORIENTED_EDGE('',*,*,#1750,.T.);
#2241=ORIENTED_EDGE('',*,*,#1751,.T.);
#2242=ORIENTED_EDGE('',*,*,#1748,.F.);
#2243=ORIENTED_EDGE('',*,*,#1674,.F.);
#2244=ORIENTED_EDGE('',*,*,#1707,.T.);
#2245=ORIENTED_EDGE('',*,*,#1752,.F.);
#2246=ORIENTED_EDGE('',*,*,#1696,.F.);
#2247=ORIENTED_EDGE('',*,*,#1753,.T.);
#2248=ORIENTED_EDGE('',*,*,#1706,.T.);
#2249=ORIENTED_EDGE('',*,*,#1754,.F.);
#2250=ORIENTED_EDGE('',*,*,#1697,.F.);
#2251=ORIENTED_EDGE('',*,*,#1752,.T.);
#2252=ORIENTED_EDGE('',*,*,#1755,.T.);
#2253=ORIENTED_EDGE('',*,*,#1756,.T.);
#2254=ORIENTED_EDGE('',*,*,#1757,.F.);
#2255=ORIENTED_EDGE('',*,*,#1698,.F.);
#2256=ORIENTED_EDGE('',*,*,#1754,.T.);
#2257=ORIENTED_EDGE('',*,*,#1705,.T.);
#2258=ORIENTED_EDGE('',*,*,#1758,.F.);
#2259=ORIENTED_EDGE('',*,*,#1759,.F.);
#2260=ORIENTED_EDGE('',*,*,#1760,.T.);
#2261=ORIENTED_EDGE('',*,*,#1761,.T.);
#2262=ORIENTED_EDGE('',*,*,#1699,.F.);
#2263=ORIENTED_EDGE('',*,*,#1757,.T.);
#2264=ORIENTED_EDGE('',*,*,#1762,.F.);
#2265=ORIENTED_EDGE('',*,*,#1758,.T.);
#2266=ORIENTED_EDGE('',*,*,#1704,.T.);
#2267=ORIENTED_EDGE('',*,*,#1763,.T.);
#2268=ORIENTED_EDGE('',*,*,#1764,.F.);
#2269=ORIENTED_EDGE('',*,*,#1765,.F.);
#2270=ORIENTED_EDGE('',*,*,#1766,.F.);
#2271=ORIENTED_EDGE('',*,*,#1767,.T.);
#2272=ORIENTED_EDGE('',*,*,#1671,.F.);
#2273=ORIENTED_EDGE('',*,*,#1768,.T.);
#2274=ORIENTED_EDGE('',*,*,#1673,.F.);
#2275=ORIENTED_EDGE('',*,*,#1769,.T.);
#2276=ORIENTED_EDGE('',*,*,#1770,.T.);
#2277=ORIENTED_EDGE('',*,*,#1771,.F.);
#2278=ORIENTED_EDGE('',*,*,#1772,.F.);
#2279=ORIENTED_EDGE('',*,*,#1773,.T.);
#2280=ORIENTED_EDGE('',*,*,#1701,.T.);
#2281=ORIENTED_EDGE('',*,*,#1668,.F.);
#2282=ORIENTED_EDGE('',*,*,#1774,.T.);
#2283=ORIENTED_EDGE('',*,*,#1750,.F.);
#2284=ORIENTED_EDGE('',*,*,#1727,.T.);
#2285=ORIENTED_EDGE('',*,*,#1744,.F.);
#2286=ORIENTED_EDGE('',*,*,#1676,.F.);
#2287=ORIENTED_EDGE('',*,*,#1747,.T.);
#2288=ORIENTED_EDGE('',*,*,#1695,.F.);
#2289=ORIENTED_EDGE('',*,*,#1775,.T.);
#2290=ORIENTED_EDGE('',*,*,#1708,.T.);
#2291=ORIENTED_EDGE('',*,*,#1753,.F.);
#2292=ORIENTED_EDGE('',*,*,#1709,.F.);
#2293=ORIENTED_EDGE('',*,*,#1775,.F.);
#2294=ORIENTED_EDGE('',*,*,#1694,.T.);
#2295=ORIENTED_EDGE('',*,*,#1746,.F.);
#2296=ORIENTED_EDGE('',*,*,#1725,.F.);
#2297=ORIENTED_EDGE('',*,*,#1742,.F.);
#2298=ORIENTED_EDGE('',*,*,#1678,.T.);
#2299=ORIENTED_EDGE('',*,*,#1743,.F.);
#2300=ORIENTED_EDGE('',*,*,#1723,.F.);
#2301=ORIENTED_EDGE('',*,*,#1740,.F.);
#2302=ORIENTED_EDGE('',*,*,#1680,.T.);
#2303=ORIENTED_EDGE('',*,*,#1741,.F.);
#2304=ORIENTED_EDGE('',*,*,#1721,.F.);
#2305=ORIENTED_EDGE('',*,*,#1738,.F.);
#2306=ORIENTED_EDGE('',*,*,#1682,.T.);
#2307=ORIENTED_EDGE('',*,*,#1739,.F.);
#2308=ORIENTED_EDGE('',*,*,#1719,.F.);
#2309=ORIENTED_EDGE('',*,*,#1736,.F.);
#2310=ORIENTED_EDGE('',*,*,#1684,.T.);
#2311=ORIENTED_EDGE('',*,*,#1737,.F.);
#2312=ORIENTED_EDGE('',*,*,#1717,.F.);
#2313=ORIENTED_EDGE('',*,*,#1734,.F.);
#2314=ORIENTED_EDGE('',*,*,#1686,.T.);
#2315=ORIENTED_EDGE('',*,*,#1735,.F.);
#2316=ORIENTED_EDGE('',*,*,#1715,.F.);
#2317=ORIENTED_EDGE('',*,*,#1732,.F.);
#2318=ORIENTED_EDGE('',*,*,#1688,.T.);
#2319=ORIENTED_EDGE('',*,*,#1733,.F.);
#2320=ORIENTED_EDGE('',*,*,#1713,.F.);
#2321=ORIENTED_EDGE('',*,*,#1730,.F.);
#2322=ORIENTED_EDGE('',*,*,#1690,.T.);
#2323=ORIENTED_EDGE('',*,*,#1731,.F.);
#2324=ORIENTED_EDGE('',*,*,#1711,.F.);
#2325=ORIENTED_EDGE('',*,*,#1745,.F.);
#2326=ORIENTED_EDGE('',*,*,#1692,.T.);
#2327=ORIENTED_EDGE('',*,*,#1729,.F.);
#2328=ORIENTED_EDGE('',*,*,#1776,.T.);
#2329=ORIENTED_EDGE('',*,*,#1774,.F.);
#2330=ORIENTED_EDGE('',*,*,#1777,.F.);
#2331=ORIENTED_EDGE('',*,*,#1762,.T.);
#2332=ORIENTED_EDGE('',*,*,#1778,.T.);
#2333=ORIENTED_EDGE('',*,*,#1755,.F.);
#2334=ORIENTED_EDGE('',*,*,#1779,.F.);
#2335=ORIENTED_EDGE('',*,*,#1749,.T.);
#2336=ORIENTED_EDGE('',*,*,#1667,.T.);
#2337=ORIENTED_EDGE('',*,*,#1779,.T.);
#2338=ORIENTED_EDGE('',*,*,#1759,.T.);
#2339=ORIENTED_EDGE('',*,*,#1777,.T.);
#2340=ORIENTED_EDGE('',*,*,#1659,.F.);
#2341=ORIENTED_EDGE('',*,*,#1751,.F.);
#2342=ORIENTED_EDGE('',*,*,#1776,.F.);
#2343=ORIENTED_EDGE('',*,*,#1756,.F.);
#2344=ORIENTED_EDGE('',*,*,#1778,.F.);
#2345=ORIENTED_EDGE('',*,*,#1660,.T.);
#2346=ORIENTED_EDGE('',*,*,#1770,.F.);
#2347=ORIENTED_EDGE('',*,*,#1780,.T.);
#2348=ORIENTED_EDGE('',*,*,#1766,.T.);
#2349=ORIENTED_EDGE('',*,*,#1781,.T.);
#2350=ORIENTED_EDGE('',*,*,#1760,.F.);
#2351=ORIENTED_EDGE('',*,*,#1782,.F.);
#2352=ORIENTED_EDGE('',*,*,#1653,.T.);
#2353=ORIENTED_EDGE('',*,*,#1665,.F.);
#2354=ORIENTED_EDGE('',*,*,#1783,.T.);
#2355=ORIENTED_EDGE('',*,*,#1772,.T.);
#2356=ORIENTED_EDGE('',*,*,#1784,.T.);
#2357=ORIENTED_EDGE('',*,*,#1764,.T.);
#2358=ORIENTED_EDGE('',*,*,#1785,.T.);
#2359=ORIENTED_EDGE('',*,*,#1654,.F.);
#2360=ORIENTED_EDGE('',*,*,#1765,.T.);
#2361=ORIENTED_EDGE('',*,*,#1784,.F.);
#2362=ORIENTED_EDGE('',*,*,#1771,.T.);
#2363=ORIENTED_EDGE('',*,*,#1782,.T.);
#2364=ORIENTED_EDGE('',*,*,#1672,.F.);
#2365=ORIENTED_EDGE('',*,*,#1767,.F.);
#2366=ORIENTED_EDGE('',*,*,#1780,.F.);
#2367=ORIENTED_EDGE('',*,*,#1769,.F.);
#2368=ORIENTED_EDGE('',*,*,#1783,.F.);
#2369=ORIENTED_EDGE('',*,*,#1664,.F.);
#2370=ORIENTED_EDGE('',*,*,#1702,.F.);
#2371=ORIENTED_EDGE('',*,*,#1773,.F.);
#2372=ORIENTED_EDGE('',*,*,#1700,.F.);
#2373=ORIENTED_EDGE('',*,*,#1761,.F.);
#2374=ORIENTED_EDGE('',*,*,#1781,.F.);
#2375=ORIENTED_EDGE('',*,*,#1768,.F.);
#2376=ORIENTED_EDGE('',*,*,#1785,.F.);
#2377=ORIENTED_EDGE('',*,*,#1763,.F.);
#2378=ORIENTED_EDGE('',*,*,#1703,.F.);
#2379=ORIENTED_EDGE('',*,*,#1666,.F.);
#3028=CYLINDRICAL_SURFACE('',#3356,2.);
#3029=CYLINDRICAL_SURFACE('',#3359,2.);
#3030=CYLINDRICAL_SURFACE('',#3362,2.);
#3031=CYLINDRICAL_SURFACE('',#3365,2.);
#3032=CYLINDRICAL_SURFACE('',#3413,1.);
#3033=CYLINDRICAL_SURFACE('',#3414,1.);
#3034=CYLINDRICAL_SURFACE('',#3415,1.);
#3035=CYLINDRICAL_SURFACE('',#3416,1.);
#3036=CYLINDRICAL_SURFACE('',#3417,1.);
#3037=CYLINDRICAL_SURFACE('',#3418,1.);
#3038=CYLINDRICAL_SURFACE('',#3419,1.);
#3039=CYLINDRICAL_SURFACE('',#3420,1.);
#3040=CYLINDRICAL_SURFACE('',#3421,1.);
#3041=CYLINDRICAL_SURFACE('',#3433,3.5);
#3042=CYLINDRICAL_SURFACE('',#3434,3.5);
#3043=CYLINDRICAL_SURFACE('',#3435,3.5);
#3044=CYLINDRICAL_SURFACE('',#3436,3.5);
#3091=ADVANCED_FACE('',(#242),#3028,.F.);
#3092=ADVANCED_FACE('',(#243),#3029,.F.);
#3093=ADVANCED_FACE('',(#244),#3030,.F.);
#3094=ADVANCED_FACE('',(#245),#3031,.F.);
#3095=ADVANCED_FACE('',(#246),#137,.F.);
#3096=ADVANCED_FACE('',(#247),#138,.F.);
#3097=ADVANCED_FACE('',(#248,#113,#114),#139,.F.);
#3098=ADVANCED_FACE('',(#249,#115,#116),#140,.T.);
#3099=ADVANCED_FACE('',(#250),#141,.F.);
#3100=ADVANCED_FACE('',(#251),#142,.F.);
#3101=ADVANCED_FACE('',(#252),#143,.F.);
#3102=ADVANCED_FACE('',(#253),#144,.F.);
#3103=ADVANCED_FACE('',(#254),#145,.F.);
#3104=ADVANCED_FACE('',(#255),#146,.F.);
#3105=ADVANCED_FACE('',(#256),#147,.F.);
#3106=ADVANCED_FACE('',(#257),#148,.F.);
#3107=ADVANCED_FACE('',(#258),#149,.F.);
#3108=ADVANCED_FACE('',(#259),#150,.F.);
#3109=ADVANCED_FACE('',(#260),#151,.F.);
#3110=ADVANCED_FACE('',(#261),#152,.F.);
#3111=ADVANCED_FACE('',(#262),#153,.F.);
#3112=ADVANCED_FACE('',(#263),#154,.F.);
#3113=ADVANCED_FACE('',(#264),#155,.F.);
#3114=ADVANCED_FACE('',(#265),#156,.F.);
#3115=ADVANCED_FACE('',(#266),#157,.F.);
#3116=ADVANCED_FACE('',(#267),#158,.F.);
#3117=ADVANCED_FACE('',(#268),#159,.F.);
#3118=ADVANCED_FACE('',(#269),#3032,.F.);
#3119=ADVANCED_FACE('',(#270),#3033,.F.);
#3120=ADVANCED_FACE('',(#271),#3034,.F.);
#3121=ADVANCED_FACE('',(#272),#3035,.F.);
#3122=ADVANCED_FACE('',(#273),#3036,.F.);
#3123=ADVANCED_FACE('',(#274),#3037,.F.);
#3124=ADVANCED_FACE('',(#275),#3038,.F.);
#3125=ADVANCED_FACE('',(#276),#3039,.F.);
#3126=ADVANCED_FACE('',(#277),#3040,.F.);
#3127=ADVANCED_FACE('',(#278),#160,.F.);
#3128=ADVANCED_FACE('',(#279),#161,.F.);
#3129=ADVANCED_FACE('',(#280,#117),#162,.T.);
#3130=ADVANCED_FACE('',(#281,#118),#163,.F.);
#3131=ADVANCED_FACE('',(#282,#119),#164,.F.);
#3132=ADVANCED_FACE('',(#283,#120),#165,.T.);
#3133=ADVANCED_FACE('',(#284),#166,.T.);
#3134=ADVANCED_FACE('',(#285),#3041,.T.);
#3135=ADVANCED_FACE('',(#286),#3042,.T.);
#3136=ADVANCED_FACE('',(#287),#3043,.T.);
#3137=ADVANCED_FACE('',(#288),#3044,.T.);
#3269=CLOSED_SHELL('',(#3091,#3092,#3093,#3094,#3095,#3096,#3097,#3098,
#3099,#3100,#3101,#3102,#3103,#3104,#3105,#3106,#3107,#3108,#3109,#3110,
#3111,#3112,#3113,#3114,#3115,#3116,#3117,#3118,#3119,#3120,#3121,#3122,
#3123,#3124,#3125,#3126,#3127,#3128,#3129,#3130,#3131,#3132,#3133,#3134,
#3135,#3136,#3137));
#3355=AXIS2_PLACEMENT_3D('',#4651,#3687,#3688);
#3356=AXIS2_PLACEMENT_3D('',#4652,#3689,#3690);
#3357=AXIS2_PLACEMENT_3D('',#4654,#3691,#3692);
#3358=AXIS2_PLACEMENT_3D('',#4657,#3694,#3695);
#3359=AXIS2_PLACEMENT_3D('',#4658,#3696,#3697);
#3360=AXIS2_PLACEMENT_3D('',#4660,#3698,#3699);
#3361=AXIS2_PLACEMENT_3D('',#4663,#3701,#3702);
#3362=AXIS2_PLACEMENT_3D('',#4664,#3703,#3704);
#3363=AXIS2_PLACEMENT_3D('',#4666,#3705,#3706);
#3364=AXIS2_PLACEMENT_3D('',#4669,#3708,#3709);
#3365=AXIS2_PLACEMENT_3D('',#4670,#3710,#3711);
#3366=AXIS2_PLACEMENT_3D('',#4672,#3712,#3713);
#3367=AXIS2_PLACEMENT_3D('',#4675,#3715,#3716);
#3368=AXIS2_PLACEMENT_3D('',#4676,#3717,#3718);
#3369=AXIS2_PLACEMENT_3D('',#4685,#3723,#3724);
#3370=AXIS2_PLACEMENT_3D('',#4694,#3729,#3730);
#3371=AXIS2_PLACEMENT_3D('',#4699,#3732,#3733);
#3372=AXIS2_PLACEMENT_3D('',#4711,#3739,#3740);
#3373=AXIS2_PLACEMENT_3D('',#4715,#3742,#3743);
#3374=AXIS2_PLACEMENT_3D('',#4719,#3745,#3746);
#3375=AXIS2_PLACEMENT_3D('',#4723,#3748,#3749);
#3376=AXIS2_PLACEMENT_3D('',#4727,#3751,#3752);
#3377=AXIS2_PLACEMENT_3D('',#4731,#3754,#3755);
#3378=AXIS2_PLACEMENT_3D('',#4735,#3757,#3758);
#3379=AXIS2_PLACEMENT_3D('',#4739,#3760,#3761);
#3380=AXIS2_PLACEMENT_3D('',#4743,#3763,#3764);
#3381=AXIS2_PLACEMENT_3D('',#4754,#3770,#3771);
#3382=AXIS2_PLACEMENT_3D('',#4755,#3772,#3773);
#3383=AXIS2_PLACEMENT_3D('',#4758,#3775,#3776);
#3384=AXIS2_PLACEMENT_3D('',#4760,#3777,#3778);
#3385=AXIS2_PLACEMENT_3D('',#4772,#3784,#3785);
#3386=AXIS2_PLACEMENT_3D('',#4776,#3787,#3788);
#3387=AXIS2_PLACEMENT_3D('',#4780,#3790,#3791);
#3388=AXIS2_PLACEMENT_3D('',#4784,#3793,#3794);
#3389=AXIS2_PLACEMENT_3D('',#4788,#3796,#3797);
#3390=AXIS2_PLACEMENT_3D('',#4792,#3799,#3800);
#3391=AXIS2_PLACEMENT_3D('',#4796,#3802,#3803);
#3392=AXIS2_PLACEMENT_3D('',#4800,#3805,#3806);
#3393=AXIS2_PLACEMENT_3D('',#4804,#3808,#3809);
#3394=AXIS2_PLACEMENT_3D('',#4810,#3813,#3814);
#3395=AXIS2_PLACEMENT_3D('',#4813,#3817,#3818);
#3396=AXIS2_PLACEMENT_3D('',#4816,#3821,#3822);
#3397=AXIS2_PLACEMENT_3D('',#4819,#3825,#3826);
#3398=AXIS2_PLACEMENT_3D('',#4822,#3829,#3830);
#3399=AXIS2_PLACEMENT_3D('',#4825,#3833,#3834);
#3400=AXIS2_PLACEMENT_3D('',#4828,#3837,#3838);
#3401=AXIS2_PLACEMENT_3D('',#4831,#3841,#3842);
#3402=AXIS2_PLACEMENT_3D('',#4834,#3845,#3846);
#3403=AXIS2_PLACEMENT_3D('',#4837,#3849,#3850);
#3404=AXIS2_PLACEMENT_3D('',#4842,#3854,#3855);
#3405=AXIS2_PLACEMENT_3D('',#4846,#3858,#3859);
#3406=AXIS2_PLACEMENT_3D('',#4849,#3862,#3863);
#3407=AXIS2_PLACEMENT_3D('',#4851,#3865,#3866);
#3408=AXIS2_PLACEMENT_3D('',#4861,#3872,#3873);
#3409=AXIS2_PLACEMENT_3D('',#4872,#3880,#3881);
#3410=AXIS2_PLACEMENT_3D('',#4878,#3885,#3886);
#3411=AXIS2_PLACEMENT_3D('',#4889,#3893,#3894);
#3412=AXIS2_PLACEMENT_3D('',#4890,#3895,#3896);
#3413=AXIS2_PLACEMENT_3D('',#4892,#3898,#3899);
#3414=AXIS2_PLACEMENT_3D('',#4893,#3900,#3901);
#3415=AXIS2_PLACEMENT_3D('',#4894,#3902,#3903);
#3416=AXIS2_PLACEMENT_3D('',#4895,#3904,#3905);
#3417=AXIS2_PLACEMENT_3D('',#4896,#3906,#3907);
#3418=AXIS2_PLACEMENT_3D('',#4897,#3908,#3909);
#3419=AXIS2_PLACEMENT_3D('',#4898,#3910,#3911);
#3420=AXIS2_PLACEMENT_3D('',#4899,#3912,#3913);
#3421=AXIS2_PLACEMENT_3D('',#4900,#3914,#3915);
#3422=AXIS2_PLACEMENT_3D('',#4901,#3916,#3917);
#3423=AXIS2_PLACEMENT_3D('',#4904,#3920,#3921);
#3424=AXIS2_PLACEMENT_3D('',#4907,#3924,#3925);
#3425=AXIS2_PLACEMENT_3D('',#4908,#3926,#3927);
#3426=AXIS2_PLACEMENT_3D('',#4909,#3928,#3929);
#3427=AXIS2_PLACEMENT_3D('',#4910,#3930,#3931);
#3428=AXIS2_PLACEMENT_3D('',#4911,#3932,#3933);
#3429=AXIS2_PLACEMENT_3D('',#4913,#3935,#3936);
#3430=AXIS2_PLACEMENT_3D('',#4914,#3937,#3938);
#3431=AXIS2_PLACEMENT_3D('',#4916,#3940,#3941);
#3432=AXIS2_PLACEMENT_3D('',#4917,#3942,#3943);
#3433=AXIS2_PLACEMENT_3D('',#4918,#3944,#3945);
#3434=AXIS2_PLACEMENT_3D('',#4919,#3946,#3947);
#3435=AXIS2_PLACEMENT_3D('',#4920,#3948,#3949);
#3436=AXIS2_PLACEMENT_3D('',#4921,#3950,#3951);
#3687=DIRECTION('axis',(0.,0.,1.));
#3688=DIRECTION('refdir',(1.,0.,0.));
#3689=DIRECTION('center_axis',(0.,0.,-1.));
#3690=DIRECTION('ref_axis',(-1.,0.,0.));
#3691=DIRECTION('center_axis',(0.,0.,-1.));
#3692=DIRECTION('ref_axis',(-1.,0.,0.));
#3693=DIRECTION('',(0.,0.,-1.));
#3694=DIRECTION('center_axis',(5.55111512312578E-17,2.47817639425258E-17,
1.));
#3695=DIRECTION('ref_axis',(1.,-1.37566424599088E-33,-5.55111512312578E-17));
#3696=DIRECTION('center_axis',(0.,0.,-1.));
#3697=DIRECTION('ref_axis',(-1.,0.,0.));
#3698=DIRECTION('center_axis',(5.55111512312578E-17,2.47817639425258E-17,
1.));
#3699=DIRECTION('ref_axis',(1.,-1.37566424599088E-33,-5.55111512312578E-17));
#3700=DIRECTION('',(0.,0.,-1.));
#3701=DIRECTION('center_axis',(0.,0.,-1.));
#3702=DIRECTION('ref_axis',(-1.,0.,0.));
#3703=DIRECTION('center_axis',(0.,0.,1.));
#3704=DIRECTION('ref_axis',(1.,0.,0.));
#3705=DIRECTION('center_axis',(0.,0.,1.));
#3706=DIRECTION('ref_axis',(1.,0.,0.));
#3707=DIRECTION('',(0.,0.,1.));
#3708=DIRECTION('center_axis',(0.,0.,1.));
#3709=DIRECTION('ref_axis',(1.,0.,0.));
#3710=DIRECTION('center_axis',(0.,0.,1.));
#3711=DIRECTION('ref_axis',(1.,0.,0.));
#3712=DIRECTION('center_axis',(0.,0.,1.));
#3713=DIRECTION('ref_axis',(1.,0.,0.));
#3714=DIRECTION('',(0.,0.,1.));
#3715=DIRECTION('center_axis',(0.,0.,1.));
#3716=DIRECTION('ref_axis',(1.,0.,0.));
#3717=DIRECTION('center_axis',(0.,1.,0.));
#3718=DIRECTION('ref_axis',(0.,0.,1.));
#3719=DIRECTION('',(1.,0.,0.));
#3720=DIRECTION('',(0.,0.,1.));
#3721=DIRECTION('',(-1.,1.79745021839835E-17,5.55111512312578E-17));
#3722=DIRECTION('',(0.,0.,-1.));
#3723=DIRECTION('center_axis',(-0.766044443118972,-0.642787609686546,0.));
#3724=DIRECTION('ref_axis',(0.642787609686546,-0.766044443118972,0.));
#3725=DIRECTION('',(-0.642787609686546,0.766044443118972,0.));
#3726=DIRECTION('',(0.,0.,-1.));
#3727=DIRECTION('',(-0.642787609686546,0.766044443118972,0.));
#3728=DIRECTION('',(0.,0.,-1.));
#3729=DIRECTION('center_axis',(0.,0.,-1.));
#3730=DIRECTION('ref_axis',(-1.,0.,0.));
#3731=DIRECTION('',(1.,0.,0.));
#3732=DIRECTION('center_axis',(0.,0.,1.));
#3733=DIRECTION('ref_axis',(-1.,0.,0.));
#3734=DIRECTION('',(-8.47613560090905E-17,1.,0.));
#3735=DIRECTION('',(-0.642787609686546,0.766044443118972,0.));
#3736=DIRECTION('',(0.,1.,0.));
#3737=DIRECTION('',(1.,0.,0.));
#3738=DIRECTION('',(-1.23908819712629E-16,1.,0.));
#3739=DIRECTION('center_axis',(0.,0.,1.));
#3740=DIRECTION('ref_axis',(1.,0.,0.));
#3741=DIRECTION('',(-1.23908819712629E-16,1.,0.));
#3742=DIRECTION('center_axis',(0.,0.,1.));
#3743=DIRECTION('ref_axis',(1.,0.,0.));
#3744=DIRECTION('',(-1.23908819712629E-16,1.,0.));
#3745=DIRECTION('center_axis',(0.,0.,1.));
#3746=DIRECTION('ref_axis',(1.,0.,0.));
#3747=DIRECTION('',(-1.23908819712629E-16,1.,0.));
#3748=DIRECTION('center_axis',(0.,0.,1.));
#3749=DIRECTION('ref_axis',(1.,0.,0.));
#3750=DIRECTION('',(-1.23908819712629E-16,1.,0.));
#3751=DIRECTION('center_axis',(0.,0.,1.));
#3752=DIRECTION('ref_axis',(1.,0.,0.));
#3753=DIRECTION('',(-1.23908819712629E-16,1.,0.));
#3754=DIRECTION('center_axis',(0.,0.,1.));
#3755=DIRECTION('ref_axis',(1.,0.,0.));
#3756=DIRECTION('',(-1.23908819712629E-16,1.,0.));
#3757=DIRECTION('center_axis',(0.,0.,1.));
#3758=DIRECTION('ref_axis',(1.,0.,0.));
#3759=DIRECTION('',(-1.23908819712629E-16,1.,0.));
#3760=DIRECTION('center_axis',(0.,0.,1.));
#3761=DIRECTION('ref_axis',(1.,0.,0.));
#3762=DIRECTION('',(-1.23908819712629E-16,1.,0.));
#3763=DIRECTION('center_axis',(0.,0.,1.));
#3764=DIRECTION('ref_axis',(1.,0.,0.));
#3765=DIRECTION('',(-1.23908819712629E-16,1.,0.));
#3766=DIRECTION('',(-1.,0.,0.));
#3767=DIRECTION('',(-0.258819045102514,-0.96592582628907,0.));
#3768=DIRECTION('',(0.642787609686546,-0.766044443118972,0.));
#3769=DIRECTION('',(-4.47692281884469E-17,-1.,0.));
#3770=DIRECTION('center_axis',(0.,0.,1.));
#3771=DIRECTION('ref_axis',(-1.,0.,0.));
#3772=DIRECTION('center_axis',(0.,0.,-1.));
#3773=DIRECTION('ref_axis',(-1.,0.,0.));
#3774=DIRECTION('',(-8.47613560090905E-17,1.,0.));
#3775=DIRECTION('center_axis',(0.,0.,-1.));
#3776=DIRECTION('ref_axis',(-1.,0.,0.));
#3777=DIRECTION('center_axis',(0.,0.,-1.));
#3778=DIRECTION('ref_axis',(-1.,0.,0.));
#3779=DIRECTION('',(-4.47692281884469E-17,-1.,0.));
#3780=DIRECTION('',(0.642787609686546,-0.766044443118972,0.));
#3781=DIRECTION('',(-0.258819045102514,-0.96592582628907,0.));
#3782=DIRECTION('',(-1.,0.,0.));
#3783=DIRECTION('',(-1.23908819712629E-16,1.,0.));
#3784=DIRECTION('center_axis',(0.,0.,1.));
#3785=DIRECTION('ref_axis',(1.,0.,0.));
#3786=DIRECTION('',(-1.23908819712629E-16,1.,0.));
#3787=DIRECTION('center_axis',(0.,0.,1.));
#3788=DIRECTION('ref_axis',(1.,0.,0.));
#3789=DIRECTION('',(-1.23908819712629E-16,1.,0.));
#3790=DIRECTION('center_axis',(0.,0.,1.));
#3791=DIRECTION('ref_axis',(1.,0.,0.));
#3792=DIRECTION('',(-1.23908819712629E-16,1.,0.));
#3793=DIRECTION('center_axis',(0.,0.,1.));
#3794=DIRECTION('ref_axis',(1.,0.,0.));
#3795=DIRECTION('',(-1.23908819712629E-16,1.,0.));
#3796=DIRECTION('center_axis',(0.,0.,1.));
#3797=DIRECTION('ref_axis',(1.,0.,0.));
#3798=DIRECTION('',(-1.23908819712629E-16,1.,0.));
#3799=DIRECTION('center_axis',(0.,0.,1.));
#3800=DIRECTION('ref_axis',(1.,0.,0.));
#3801=DIRECTION('',(-1.23908819712629E-16,1.,0.));
#3802=DIRECTION('center_axis',(0.,0.,1.));
#3803=DIRECTION('ref_axis',(1.,0.,0.));
#3804=DIRECTION('',(-1.23908819712629E-16,1.,0.));
#3805=DIRECTION('center_axis',(0.,0.,1.));
#3806=DIRECTION('ref_axis',(1.,0.,0.));
#3807=DIRECTION('',(-1.23908819712629E-16,1.,0.));
#3808=DIRECTION('center_axis',(0.,0.,1.));
#3809=DIRECTION('ref_axis',(1.,0.,0.));
#3810=DIRECTION('',(-1.23908819712629E-16,1.,0.));
#3811=DIRECTION('',(1.,0.,0.));
#3812=DIRECTION('',(0.,1.,0.));
#3813=DIRECTION('center_axis',(-1.,-1.23908819712629E-16,0.));
#3814=DIRECTION('ref_axis',(1.23908819712629E-16,-1.,0.));
#3815=DIRECTION('',(0.,0.,1.));
#3816=DIRECTION('',(0.,0.,-1.));
#3817=DIRECTION('center_axis',(-1.,-1.23908819712629E-16,0.));
#3818=DIRECTION('ref_axis',(1.23908819712629E-16,-1.,0.));
#3819=DIRECTION('',(0.,0.,1.));
#3820=DIRECTION('',(0.,0.,-1.));
#3821=DIRECTION('center_axis',(-1.,-1.23908819712629E-16,0.));
#3822=DIRECTION('ref_axis',(1.23908819712629E-16,-1.,0.));
#3823=DIRECTION('',(0.,0.,1.));
#3824=DIRECTION('',(0.,0.,-1.));
#3825=DIRECTION('center_axis',(-1.,-1.23908819712629E-16,0.));
#3826=DIRECTION('ref_axis',(1.23908819712629E-16,-1.,0.));
#3827=DIRECTION('',(0.,0.,1.));
#3828=DIRECTION('',(0.,0.,-1.));
#3829=DIRECTION('center_axis',(-1.,-1.23908819712629E-16,0.));
#3830=DIRECTION('ref_axis',(1.23908819712629E-16,-1.,0.));
#3831=DIRECTION('',(0.,0.,1.));
#3832=DIRECTION('',(0.,0.,-1.));
#3833=DIRECTION('center_axis',(-1.,-1.23908819712629E-16,0.));
#3834=DIRECTION('ref_axis',(1.23908819712629E-16,-1.,0.));
#3835=DIRECTION('',(0.,0.,1.));
#3836=DIRECTION('',(0.,0.,-1.));
#3837=DIRECTION('center_axis',(-1.,-1.23908819712629E-16,0.));
#3838=DIRECTION('ref_axis',(1.23908819712629E-16,-1.,0.));
#3839=DIRECTION('',(0.,0.,1.));
#3840=DIRECTION('',(0.,0.,-1.));
#3841=DIRECTION('center_axis',(-1.,-1.23908819712629E-16,0.));
#3842=DIRECTION('ref_axis',(1.23908819712629E-16,-1.,0.));
#3843=DIRECTION('',(0.,0.,1.));
#3844=DIRECTION('',(0.,0.,-1.));
#3845=DIRECTION('center_axis',(-1.,-1.23908819712629E-16,0.));
#3846=DIRECTION('ref_axis',(1.23908819712629E-16,-1.,0.));
#3847=DIRECTION('',(0.,0.,-1.));
#3848=DIRECTION('',(0.,0.,1.));
#3849=DIRECTION('center_axis',(-1.,0.,0.));
#3850=DIRECTION('ref_axis',(0.,0.,1.));
#3851=DIRECTION('',(0.,0.,-1.));
#3852=DIRECTION('',(0.,0.,-1.));
#3853=DIRECTION('',(0.,0.,1.));
#3854=DIRECTION('center_axis',(-0.766044443118972,-0.642787609686546,0.));
#3855=DIRECTION('ref_axis',(0.642787609686546,-0.766044443118972,0.));
#3856=DIRECTION('',(0.,0.,-1.));
#3857=DIRECTION('',(-0.642787609686546,0.766044443118972,0.));
#3858=DIRECTION('center_axis',(0.,-1.,0.));
#3859=DIRECTION('ref_axis',(0.,0.,-1.));
#3860=DIRECTION('',(0.,0.,-1.));
#3861=DIRECTION('',(0.,0.,-1.));
#3862=DIRECTION('center_axis',(0.96592582628907,-0.258819045102514,0.));
#3863=DIRECTION('ref_axis',(0.258819045102514,0.96592582628907,0.));
#3864=DIRECTION('',(0.,0.,-1.));
#3865=DIRECTION('center_axis',(0.766044443118972,0.642787609686546,0.));
#3866=DIRECTION('ref_axis',(-0.642787609686546,0.766044443118972,0.));
#3867=DIRECTION('',(0.,0.,1.));
#3868=DIRECTION('',(0.642787609686546,-0.766044443118972,0.));
#3869=DIRECTION('',(0.,0.,-1.));
#3870=DIRECTION('',(0.,0.,-1.));
#3871=DIRECTION('',(0.642787609686546,-0.766044443118972,0.));
#3872=DIRECTION('center_axis',(1.,-4.47692281884469E-17,0.));
#3873=DIRECTION('ref_axis',(4.47692281884469E-17,1.,0.));
#3874=DIRECTION('',(-4.47692281884469E-17,-1.,2.47817639425258E-17));
#3875=DIRECTION('',(0.,0.,1.));
#3876=DIRECTION('',(0.,0.,1.));
#3877=DIRECTION('',(0.,0.,1.));
#3878=DIRECTION('',(-4.47692281884469E-17,-1.,2.47817639425258E-17));
#3879=DIRECTION('',(0.,0.,-1.));
#3880=DIRECTION('center_axis',(0.,1.,0.));
#3881=DIRECTION('ref_axis',(0.,0.,1.));
#3882=DIRECTION('',(-1.,1.79745021839835E-17,5.55111512312578E-17));
#3883=DIRECTION('',(0.,0.,1.));
#3884=DIRECTION('',(0.,0.,-1.));
#3885=DIRECTION('center_axis',(-1.,-8.47613560090905E-17,0.));
#3886=DIRECTION('ref_axis',(8.47613560090905E-17,-1.,0.));
#3887=DIRECTION('',(0.,0.,-1.));
#3888=DIRECTION('',(1.79745021839835E-17,1.,-2.47817639425258E-17));
#3889=DIRECTION('',(5.55111512312578E-17,-9.97785309041681E-34,1.));
#3890=DIRECTION('',(1.79745021839835E-17,1.,-2.47817639425258E-17));
#3891=DIRECTION('',(0.,0.,-1.));
#3892=DIRECTION('',(0.,0.,1.));
#3893=DIRECTION('center_axis',(0.,1.,0.));
#3894=DIRECTION('ref_axis',(0.,0.,1.));
#3895=DIRECTION('center_axis',(-1.,-1.23908819712629E-16,0.));
#3896=DIRECTION('ref_axis',(1.23908819712629E-16,-1.,0.));
#3897=DIRECTION('',(0.,0.,-1.));
#3898=DIRECTION('center_axis',(0.,0.,1.));
#3899=DIRECTION('ref_axis',(-1.,1.22464679914735E-16,0.));
#3900=DIRECTION('center_axis',(0.,0.,1.));
#3901=DIRECTION('ref_axis',(-1.,1.22464679914735E-16,0.));
#3902=DIRECTION('center_axis',(0.,0.,1.));
#3903=DIRECTION('ref_axis',(-1.,1.22464679914735E-16,0.));
#3904=DIRECTION('center_axis',(0.,0.,1.));
#3905=DIRECTION('ref_axis',(-1.,1.22464679914735E-16,0.));
#3906=DIRECTION('center_axis',(0.,0.,1.));
#3907=DIRECTION('ref_axis',(-1.,1.22464679914735E-16,0.));
#3908=DIRECTION('center_axis',(0.,0.,1.));
#3909=DIRECTION('ref_axis',(-1.,1.22464679914735E-16,0.));
#3910=DIRECTION('center_axis',(0.,0.,1.));
#3911=DIRECTION('ref_axis',(-1.,1.22464679914735E-16,0.));
#3912=DIRECTION('center_axis',(0.,0.,1.));
#3913=DIRECTION('ref_axis',(-1.,1.22464679914735E-16,0.));
#3914=DIRECTION('center_axis',(0.,0.,1.));
#3915=DIRECTION('ref_axis',(-1.,1.22464679914735E-16,0.));
#3916=DIRECTION('center_axis',(0.342020143325676,-0.939692620785906,0.));
#3917=DIRECTION('ref_axis',(0.939692620785906,0.342020143325676,0.));
#3918=DIRECTION('',(0.939692620785906,0.342020143325676,0.));
#3919=DIRECTION('',(0.939692620785906,0.342020143325676,0.));
#3920=DIRECTION('center_axis',(-0.642787609686546,0.766044443118972,0.));
#3921=DIRECTION('ref_axis',(-0.766044443118972,-0.642787609686546,0.));
#3922=DIRECTION('',(-0.766044443118972,-0.642787609686546,0.));
#3923=DIRECTION('',(-0.766044443118972,-0.642787609686546,0.));
#3924=DIRECTION('center_axis',(0.,0.,1.));
#3925=DIRECTION('ref_axis',(1.,0.,0.));
#3926=DIRECTION('center_axis',(0.,0.,1.));
#3927=DIRECTION('ref_axis',(1.,0.,0.));
#3928=DIRECTION('center_axis',(5.55111512312578E-17,2.47817639425258E-17,
1.));
#3929=DIRECTION('ref_axis',(1.,0.,-5.55111512312578E-17));
#3930=DIRECTION('center_axis',(-5.55111512312578E-17,-2.47817639425258E-17,
-1.));
#3931=DIRECTION('ref_axis',(1.,-1.37566424599088E-33,-5.55111512312578E-17));
#3932=DIRECTION('center_axis',(-5.55111512312578E-17,-2.47817639425258E-17,
-1.));
#3933=DIRECTION('ref_axis',(1.,-1.37566424599088E-33,-5.55111512312578E-17));
#3934=DIRECTION('',(-1.,1.79745021839835E-17,5.55111512312578E-17));
#3935=DIRECTION('center_axis',(5.55111512312578E-17,2.47817639425258E-17,
1.));
#3936=DIRECTION('ref_axis',(1.,0.,-5.55111512312578E-17));
#3937=DIRECTION('center_axis',(5.55111512312578E-17,2.47817639425258E-17,
1.));
#3938=DIRECTION('ref_axis',(1.,-1.37566424599088E-33,-5.55111512312578E-17));
#3939=DIRECTION('',(-1.,1.79745021839835E-17,5.55111512312578E-17));
#3940=DIRECTION('center_axis',(5.55111512312578E-17,2.47817639425258E-17,
1.));
#3941=DIRECTION('ref_axis',(1.,-1.37566424599088E-33,-5.55111512312578E-17));
#3942=DIRECTION('center_axis',(-1.79745021839835E-17,-1.,0.));
#3943=DIRECTION('ref_axis',(1.,-1.79745021839835E-17,0.));
#3944=DIRECTION('center_axis',(0.,0.,-1.));
#3945=DIRECTION('ref_axis',(-1.,0.,0.));
#3946=DIRECTION('center_axis',(0.,0.,-1.));
#3947=DIRECTION('ref_axis',(-1.,0.,0.));
#3948=DIRECTION('center_axis',(0.,0.,-1.));
#3949=DIRECTION('ref_axis',(-1.,0.,0.));
#3950=DIRECTION('center_axis',(0.,0.,-1.));
#3951=DIRECTION('ref_axis',(-1.,0.,0.));
#4651=CARTESIAN_POINT('',(0.,0.,0.));
#4652=CARTESIAN_POINT('Origin',(26.,-116.5,7.));
#4653=CARTESIAN_POINT('',(28.,-116.5,7.));
#4654=CARTESIAN_POINT('Origin',(26.,-116.5,7.));
#4655=CARTESIAN_POINT('',(28.,-116.5,2.));
#4656=CARTESIAN_POINT('',(28.,-116.5,7.));
#4657=CARTESIAN_POINT('Origin',(26.,-116.5,2.));
#4658=CARTESIAN_POINT('Origin',(26.,-116.5,7.));
#4659=CARTESIAN_POINT('',(28.,-116.5,-2.));
#4660=CARTESIAN_POINT('Origin',(26.,-116.5,-2.));
#4661=CARTESIAN_POINT('',(28.,-116.5,-7.));
#4662=CARTESIAN_POINT('',(28.,-116.5,7.));
#4663=CARTESIAN_POINT('Origin',(26.,-116.5,-7.));
#4664=CARTESIAN_POINT('Origin',(5.,-15.2931109241333,-7.));
#4665=CARTESIAN_POINT('',(3.,-15.2931109241333,-7.));
#4666=CARTESIAN_POINT('Origin',(5.,-15.2931109241333,-7.));
#4667=CARTESIAN_POINT('',(3.,-15.2931109241333,-5.));
#4668=CARTESIAN_POINT('',(3.,-15.2931109241333,-7.));
#4669=CARTESIAN_POINT('Origin',(5.,-15.2931109241333,-5.));
#4670=CARTESIAN_POINT('Origin',(5.,-15.2931109241333,-7.));
#4671=CARTESIAN_POINT('',(3.,-15.2931109241333,5.));
#4672=CARTESIAN_POINT('Origin',(5.,-15.2931109241333,5.));
#4673=CARTESIAN_POINT('',(3.,-15.2931109241333,7.));
#4674=CARTESIAN_POINT('',(3.,-15.2931109241333,-7.));
#4675=CARTESIAN_POINT('Origin',(5.,-15.2931109241333,7.));
#4676=CARTESIAN_POINT('Origin',(32.,-120.,7.));
#4677=CARTESIAN_POINT('',(23.5,-120.,-7.));
#4678=CARTESIAN_POINT('',(28.5,-120.,-7.));
#4679=CARTESIAN_POINT('',(32.,-120.,-7.));
#4680=CARTESIAN_POINT('',(28.5,-120.,-2.));
#4681=CARTESIAN_POINT('',(28.5,-120.,7.));
#4682=CARTESIAN_POINT('',(23.5,-120.,-2.));
#4683=CARTESIAN_POINT('',(32.,-120.,-2.));
#4684=CARTESIAN_POINT('',(23.5,-120.,7.));
#4685=CARTESIAN_POINT('Origin',(0.,0.,7.));
#4686=CARTESIAN_POINT('',(32.,-38.136114963014,-5.));
#4687=CARTESIAN_POINT('',(0.,0.,-5.));
#4688=CARTESIAN_POINT('',(32.,-38.136114963014,-5.));
#4689=CARTESIAN_POINT('',(32.,-38.136114963014,-7.));
#4690=CARTESIAN_POINT('',(32.,-38.136114963014,7.));
#4691=CARTESIAN_POINT('',(0.,0.,-7.));
#4692=CARTESIAN_POINT('',(0.,0.,-7.));
#4693=CARTESIAN_POINT('',(0.,0.,7.));
#4694=CARTESIAN_POINT('Origin',(0.,0.,7.));
#4695=CARTESIAN_POINT('',(23.5,-120.,7.));
#4696=CARTESIAN_POINT('',(28.5,-120.,7.));
#4697=CARTESIAN_POINT('',(32.,-120.,7.));
#4698=CARTESIAN_POINT('',(32.,-116.5,7.));
#4699=CARTESIAN_POINT('Origin',(28.5,-116.5,7.));
#4700=CARTESIAN_POINT('',(32.,-38.136114963014,7.));
#4701=CARTESIAN_POINT('',(32.,-38.136114963014,7.));
#4702=CARTESIAN_POINT('',(0.,0.,7.));
#4703=CARTESIAN_POINT('',(0.,0.,7.));
#4704=CARTESIAN_POINT('',(0.,5.,7.));
#4705=CARTESIAN_POINT('',(0.,0.,7.));
#4706=CARTESIAN_POINT('',(5.,5.,7.));
#4707=CARTESIAN_POINT('',(0.,5.,7.));
#4708=CARTESIAN_POINT('',(5.,9.,7.));
#4709=CARTESIAN_POINT('',(5.,40.,7.));
#4710=CARTESIAN_POINT('',(5.,11.,7.));
#4711=CARTESIAN_POINT('Origin',(5.00000000000001,10.,7.));
#4712=CARTESIAN_POINT('',(5.,12.5,7.));
#4713=CARTESIAN_POINT('',(5.,40.,7.));
#4714=CARTESIAN_POINT('',(5.,14.5,7.));
#4715=CARTESIAN_POINT('Origin',(5.00000000000001,13.5,7.));
#4716=CARTESIAN_POINT('',(5.,16.,7.));
#4717=CARTESIAN_POINT('',(5.,40.,7.));
#4718=CARTESIAN_POINT('',(5.,18.,7.));
#4719=CARTESIAN_POINT('Origin',(5.00000000000001,17.,7.));
#4720=CARTESIAN_POINT('',(5.,19.5,7.));
#4721=CARTESIAN_POINT('',(5.,40.,7.));
#4722=CARTESIAN_POINT('',(5.,21.5,7.));
#4723=CARTESIAN_POINT('Origin',(5.00000000000001,20.5,7.));
#4724=CARTESIAN_POINT('',(5.,23.,7.));
#4725=CARTESIAN_POINT('',(5.,40.,7.));
#4726=CARTESIAN_POINT('',(5.,25.,7.));
#4727=CARTESIAN_POINT('Origin',(5.00000000000001,24.,7.));
#4728=CARTESIAN_POINT('',(5.,26.5,7.));
#4729=CARTESIAN_POINT('',(5.,40.,7.));
#4730=CARTESIAN_POINT('',(5.,28.5,7.));
#4731=CARTESIAN_POINT('Origin',(5.00000000000001,27.5,7.));
#4732=CARTESIAN_POINT('',(5.,30.,7.));
#4733=CARTESIAN_POINT('',(5.,40.,7.));
#4734=CARTESIAN_POINT('',(5.,32.,7.));
#4735=CARTESIAN_POINT('Origin',(5.00000000000001,31.,7.));
#4736=CARTESIAN_POINT('',(5.,33.5,7.));
#4737=CARTESIAN_POINT('',(5.,40.,7.));
#4738=CARTESIAN_POINT('',(5.,35.5,7.));
#4739=CARTESIAN_POINT('Origin',(5.00000000000001,34.5,7.));
#4740=CARTESIAN_POINT('',(5.,37.,7.));
#4741=CARTESIAN_POINT('',(5.,40.,7.));
#4742=CARTESIAN_POINT('',(5.,39.,7.));
#4743=CARTESIAN_POINT('Origin',(5.,38.,7.));
#4744=CARTESIAN_POINT('',(5.,40.,7.));
#4745=CARTESIAN_POINT('',(5.,40.,7.));
#4746=CARTESIAN_POINT('',(-5.,40.,7.));
#4747=CARTESIAN_POINT('',(0.,40.,7.));
#4748=CARTESIAN_POINT('',(-15.705120202908,0.0479475016143677,7.));
#4749=CARTESIAN_POINT('',(-5.,40.,7.));
#4750=CARTESIAN_POINT('',(20.,-42.5037577742085,7.));
#4751=CARTESIAN_POINT('',(-15.705120202908,0.0479475016143677,7.));
#4752=CARTESIAN_POINT('',(20.,-116.5,7.));
#4753=CARTESIAN_POINT('',(20.,-42.5037577742085,7.));
#4754=CARTESIAN_POINT('Origin',(23.5,-116.5,7.));
#4755=CARTESIAN_POINT('Origin',(0.,0.,-7.));
#4756=CARTESIAN_POINT('',(32.,-116.5,-7.));
#4757=CARTESIAN_POINT('',(32.,-38.136114963014,-7.));
#4758=CARTESIAN_POINT('Origin',(28.5,-116.5,-7.));
#4759=CARTESIAN_POINT('',(20.,-116.5,-7.));
#4760=CARTESIAN_POINT('Origin',(23.5,-116.5,-7.));
#4761=CARTESIAN_POINT('',(20.,-42.5037577742085,-7.));
#4762=CARTESIAN_POINT('',(20.,-42.5037577742085,-7.));
#4763=CARTESIAN_POINT('',(-15.705120202908,0.0479475016143677,-7.));
#4764=CARTESIAN_POINT('',(-15.705120202908,0.0479475016143677,-7.));
#4765=CARTESIAN_POINT('',(-5.,40.,-7.));
#4766=CARTESIAN_POINT('',(-5.,40.,-7.));
#4767=CARTESIAN_POINT('',(5.,40.,-7.));
#4768=CARTESIAN_POINT('',(0.,40.,-7.));
#4769=CARTESIAN_POINT('',(5.,39.,-7.));
#4770=CARTESIAN_POINT('',(5.,40.,-7.));
#4771=CARTESIAN_POINT('',(5.,37.,-7.));
#4772=CARTESIAN_POINT('Origin',(5.,38.,-7.));
#4773=CARTESIAN_POINT('',(5.,35.5,-7.));
#4774=CARTESIAN_POINT('',(5.,40.,-7.));
#4775=CARTESIAN_POINT('',(5.,33.5,-7.));
#4776=CARTESIAN_POINT('Origin',(5.00000000000001,34.5,-7.));
#4777=CARTESIAN_POINT('',(5.,32.,-7.));
#4778=CARTESIAN_POINT('',(5.,40.,-7.));
#4779=CARTESIAN_POINT('',(5.,30.,-7.));
#4780=CARTESIAN_POINT('Origin',(5.00000000000001,31.,-7.));
#4781=CARTESIAN_POINT('',(5.,28.5,-7.));
#4782=CARTESIAN_POINT('',(5.,40.,-7.));
#4783=CARTESIAN_POINT('',(5.,26.5,-7.));
#4784=CARTESIAN_POINT('Origin',(5.00000000000001,27.5,-7.));
#4785=CARTESIAN_POINT('',(5.,25.,-7.));
#4786=CARTESIAN_POINT('',(5.,40.,-7.));
#4787=CARTESIAN_POINT('',(5.,23.,-7.));
#4788=CARTESIAN_POINT('Origin',(5.00000000000001,24.,-7.));
#4789=CARTESIAN_POINT('',(5.,21.5,-7.));
#4790=CARTESIAN_POINT('',(5.,40.,-7.));
#4791=CARTESIAN_POINT('',(5.,19.5,-7.));
#4792=CARTESIAN_POINT('Origin',(5.00000000000001,20.5,-7.));
#4793=CARTESIAN_POINT('',(5.,18.,-7.));
#4794=CARTESIAN_POINT('',(5.,40.,-7.));
#4795=CARTESIAN_POINT('',(5.,16.,-7.));
#4796=CARTESIAN_POINT('Origin',(5.00000000000001,17.,-7.));
#4797=CARTESIAN_POINT('',(5.,14.5,-7.));
#4798=CARTESIAN_POINT('',(5.,40.,-7.));
#4799=CARTESIAN_POINT('',(5.,12.5,-7.));
#4800=CARTESIAN_POINT('Origin',(5.00000000000001,13.5,-7.));
#4801=CARTESIAN_POINT('',(5.,11.,-7.));
#4802=CARTESIAN_POINT('',(5.,40.,-7.));
#4803=CARTESIAN_POINT('',(5.,9.,-7.));
#4804=CARTESIAN_POINT('Origin',(5.00000000000001,10.,-7.));
#4805=CARTESIAN_POINT('',(5.,5.,-7.));
#4806=CARTESIAN_POINT('',(5.,40.,-7.));
#4807=CARTESIAN_POINT('',(0.,5.,-7.));
#4808=CARTESIAN_POINT('',(0.,5.,-7.));
#4809=CARTESIAN_POINT('',(0.,0.,-7.));
#4810=CARTESIAN_POINT('Origin',(5.,40.,7.));
#4811=CARTESIAN_POINT('',(5.,33.5,-7.));
#4812=CARTESIAN_POINT('',(5.,32.,-7.));
#4813=CARTESIAN_POINT('Origin',(5.,40.,7.));
#4814=CARTESIAN_POINT('',(5.,30.,-7.));
#4815=CARTESIAN_POINT('',(5.,28.5,-7.));
#4816=CARTESIAN_POINT('Origin',(5.,40.,7.));
#4817=CARTESIAN_POINT('',(5.,26.5,-7.));
#4818=CARTESIAN_POINT('',(5.,25.,-7.));
#4819=CARTESIAN_POINT('Origin',(5.,40.,7.));
#4820=CARTESIAN_POINT('',(5.,23.,-7.));
#4821=CARTESIAN_POINT('',(5.,21.5,-7.));
#4822=CARTESIAN_POINT('Origin',(5.,40.,7.));
#4823=CARTESIAN_POINT('',(5.,19.5,-7.));
#4824=CARTESIAN_POINT('',(5.,18.,-7.));
#4825=CARTESIAN_POINT('Origin',(5.,40.,7.));
#4826=CARTESIAN_POINT('',(5.,16.,-7.));
#4827=CARTESIAN_POINT('',(5.,14.5,-7.));
#4828=CARTESIAN_POINT('Origin',(5.,40.,7.));
#4829=CARTESIAN_POINT('',(5.,12.5,-7.));
#4830=CARTESIAN_POINT('',(5.,11.,-7.));
#4831=CARTESIAN_POINT('Origin',(5.,40.,7.));
#4832=CARTESIAN_POINT('',(5.,9.,-7.));
#4833=CARTESIAN_POINT('',(5.,5.,7.));
#4834=CARTESIAN_POINT('Origin',(5.,40.,7.));
#4835=CARTESIAN_POINT('',(5.,35.5,-7.));
#4836=CARTESIAN_POINT('',(5.,37.,-7.));
#4837=CARTESIAN_POINT('Origin',(0.,0.,7.));
#4838=CARTESIAN_POINT('',(0.,5.,7.));
#4839=CARTESIAN_POINT('',(0.,0.,5.));
#4840=CARTESIAN_POINT('',(0.,0.,7.));
#4841=CARTESIAN_POINT('',(0.,0.,-5.));
#4842=CARTESIAN_POINT('Origin',(0.,0.,7.));
#4843=CARTESIAN_POINT('',(32.,-38.136114963014,5.));
#4844=CARTESIAN_POINT('',(32.,-38.136114963014,7.));
#4845=CARTESIAN_POINT('',(32.,-38.136114963014,5.));
#4846=CARTESIAN_POINT('Origin',(0.,40.,7.));
#4847=CARTESIAN_POINT('',(-5.,40.,7.));
#4848=CARTESIAN_POINT('',(5.,40.,7.));
#4849=CARTESIAN_POINT('Origin',(-5.,40.,7.));
#4850=CARTESIAN_POINT('',(-15.705120202908,0.0479475016143677,7.));
#4851=CARTESIAN_POINT('Origin',(-15.705120202908,0.0479475016143677,7.));
#4852=CARTESIAN_POINT('',(-9.19253331742767,-7.71345131623856,-5.));
#4853=CARTESIAN_POINT('',(-9.19253331742767,-7.71345131623856,5.));
#4854=CARTESIAN_POINT('',(-9.19253331742767,-7.71345131623856,-5.));
#4855=CARTESIAN_POINT('',(20.,-42.5037577742085,5.));
#4856=CARTESIAN_POINT('',(-9.19253331742767,-7.71345131623856,5.));
#4857=CARTESIAN_POINT('',(20.,-42.5037577742085,7.));
#4858=CARTESIAN_POINT('',(20.,-42.5037577742085,-5.));
#4859=CARTESIAN_POINT('',(20.,-42.5037577742085,7.));
#4860=CARTESIAN_POINT('',(-9.19253331742767,-7.71345131623856,-5.));
#4861=CARTESIAN_POINT('Origin',(20.,-42.5037577742085,7.));
#4862=CARTESIAN_POINT('',(20.,-50.,2.));
#4863=CARTESIAN_POINT('',(20.,-116.5,2.));
#4864=CARTESIAN_POINT('',(20.,-42.5037577742085,2.));
#4865=CARTESIAN_POINT('',(20.,-116.5,7.));
#4866=CARTESIAN_POINT('',(20.,-42.5037577742085,-5.));
#4867=CARTESIAN_POINT('',(20.,-116.5,-2.));
#4868=CARTESIAN_POINT('',(20.,-116.5,7.));
#4869=CARTESIAN_POINT('',(20.,-50.,-2.));
#4870=CARTESIAN_POINT('',(20.,-42.5037577742085,-2.));
#4871=CARTESIAN_POINT('',(20.,-50.,7.));
#4872=CARTESIAN_POINT('Origin',(32.,-120.,7.));
#4873=CARTESIAN_POINT('',(28.5,-120.,2.));
#4874=CARTESIAN_POINT('',(23.5,-120.,2.));
#4875=CARTESIAN_POINT('',(32.,-120.,2.));
#4876=CARTESIAN_POINT('',(28.5,-120.,7.));
#4877=CARTESIAN_POINT('',(23.5,-120.,7.));
#4878=CARTESIAN_POINT('Origin',(32.,-38.136114963014,7.));
#4879=CARTESIAN_POINT('',(32.,-116.5,2.));
#4880=CARTESIAN_POINT('',(32.,-116.5,7.));
#4881=CARTESIAN_POINT('',(32.,-50.,2.));
#4882=CARTESIAN_POINT('',(32.,-120.,2.));
#4883=CARTESIAN_POINT('',(32.,-50.,-2.));
#4884=CARTESIAN_POINT('',(32.,-50.,-2.));
#4885=CARTESIAN_POINT('',(32.,-116.5,-2.));
#4886=CARTESIAN_POINT('',(32.,-120.,-2.));
#4887=CARTESIAN_POINT('',(32.,-116.5,7.));
#4888=CARTESIAN_POINT('',(32.,-38.136114963014,-5.));
#4889=CARTESIAN_POINT('Origin',(0.,5.,7.));
#4890=CARTESIAN_POINT('Origin',(5.,40.,7.));
#4891=CARTESIAN_POINT('',(5.,39.,-7.));
#4892=CARTESIAN_POINT('Origin',(5.,38.,-7.));
#4893=CARTESIAN_POINT('Origin',(5.00000000000001,10.,-7.));
#4894=CARTESIAN_POINT('Origin',(5.00000000000001,13.5,-7.));
#4895=CARTESIAN_POINT('Origin',(5.00000000000001,17.,-7.));
#4896=CARTESIAN_POINT('Origin',(5.00000000000001,20.5,-7.));
#4897=CARTESIAN_POINT('Origin',(5.00000000000001,24.,-7.));
#4898=CARTESIAN_POINT('Origin',(5.00000000000001,27.5,-7.));
#4899=CARTESIAN_POINT('Origin',(5.00000000000001,31.,-7.));
#4900=CARTESIAN_POINT('Origin',(5.00000000000001,34.5,-7.));
#4901=CARTESIAN_POINT('Origin',(20.,-42.5037577742085,-5.));
#4902=CARTESIAN_POINT('',(20.,-42.5037577742085,5.));
#4903=CARTESIAN_POINT('',(20.,-42.5037577742085,-5.));
#4904=CARTESIAN_POINT('Origin',(0.,0.,-5.));
#4905=CARTESIAN_POINT('',(0.,0.,5.));
#4906=CARTESIAN_POINT('',(0.,0.,-5.));
#4907=CARTESIAN_POINT('Origin',(0.,0.,-5.));
#4908=CARTESIAN_POINT('Origin',(0.,0.,5.));
#4909=CARTESIAN_POINT('Origin',(32.,-120.,2.));
#4910=CARTESIAN_POINT('Origin',(28.5,-116.5,2.));
#4911=CARTESIAN_POINT('Origin',(23.5,-116.5,2.));
#4912=CARTESIAN_POINT('',(32.,-50.,2.));
#4913=CARTESIAN_POINT('Origin',(32.,-120.,-2.));
#4914=CARTESIAN_POINT('Origin',(28.5,-116.5,-2.));
#4915=CARTESIAN_POINT('',(32.,-50.,-2.));
#4916=CARTESIAN_POINT('Origin',(23.5,-116.5,-2.));
#4917=CARTESIAN_POINT('Origin',(32.,-50.,-2.));
#4918=CARTESIAN_POINT('Origin',(28.5,-116.5,7.));
#4919=CARTESIAN_POINT('Origin',(28.5,-116.5,7.));
#4920=CARTESIAN_POINT('Origin',(23.5,-116.5,7.));
#4921=CARTESIAN_POINT('Origin',(23.5,-116.5,7.));
#5974=UNCERTAINTY_MEASURE_WITH_UNIT(LENGTH_MEASURE(0.01),#5991,
'DISTANCE_ACCURACY_VALUE',
'Maximum model space distance between geometric entities at asserted c
onnectivities');
#5981=UNCERTAINTY_MEASURE_WITH_UNIT(LENGTH_MEASURE(0.01),#5991,
'DISTANCE_ACCURACY_VALUE',
'Maximum model space distance between geometric entities at asserted c
onnectivities');
#5983=(
GEOMETRIC_REPRESENTATION_CONTEXT(3)
GLOBAL_UNCERTAINTY_ASSIGNED_CONTEXT((#5974))
GLOBAL_UNIT_ASSIGNED_CONTEXT((#5991,#5993,#5994))
REPRESENTATION_CONTEXT('','3D')
);
#5990=(
GEOMETRIC_REPRESENTATION_CONTEXT(3)
GLOBAL_UNCERTAINTY_ASSIGNED_CONTEXT((#5981))
GLOBAL_UNIT_ASSIGNED_CONTEXT((#5991,#5993,#5994))
REPRESENTATION_CONTEXT('','3D')
);
#5991=(
LENGTH_UNIT()
NAMED_UNIT(*)
SI_UNIT(.MILLI.,.METRE.)
);
#5993=(
NAMED_UNIT(*)
PLANE_ANGLE_UNIT()
SI_UNIT($,.RADIAN.)
);
#5994=(
NAMED_UNIT(*)
SI_UNIT($,.STERADIAN.)
SOLID_ANGLE_UNIT()
);
#5996=SHAPE_DEFINITION_REPRESENTATION(#6004,#6021);
#6004=PRODUCT_DEFINITION_SHAPE('',$,#6030);
#6021=SHAPE_REPRESENTATION('',(#3355),#5983);
#6028=PRODUCT_DEFINITION_CONTEXT('part definition',#6054,'design');
#6030=PRODUCT_DEFINITION('Pliers Jaw 1','Pliers Jaw 1',#6038,#6028);
#6038=PRODUCT_DEFINITION_FORMATION('',$,#6057);
#6054=APPLICATION_CONTEXT(
'Core Data for Automotive Mechanical Design Process');
#6055=PRODUCT_CONTEXT('part definition',#6054,'mechanical');
#6057=PRODUCT('Pliers Jaw 1','Pliers Jaw 1',$,(#6055));
#6065=PRESENTATION_STYLE_ASSIGNMENT((#6071));
#6071=SURFACE_STYLE_USAGE(.BOTH.,#6077);
#6077=SURFACE_SIDE_STYLE('',(#6083));
#6083=SURFACE_STYLE_FILL_AREA(#6089);
#6089=FILL_AREA_STYLE('Opaque(61,176,222)',(#6095));
#6095=FILL_AREA_STYLE_COLOUR('Opaque(61,176,222)',#6101);
#6101=COLOUR_RGB('Opaque(61,176,222)',0.23921568627451,0.690196078431373,
0.870588235294118);
ENDSEC;
END-ISO-10303-21;
